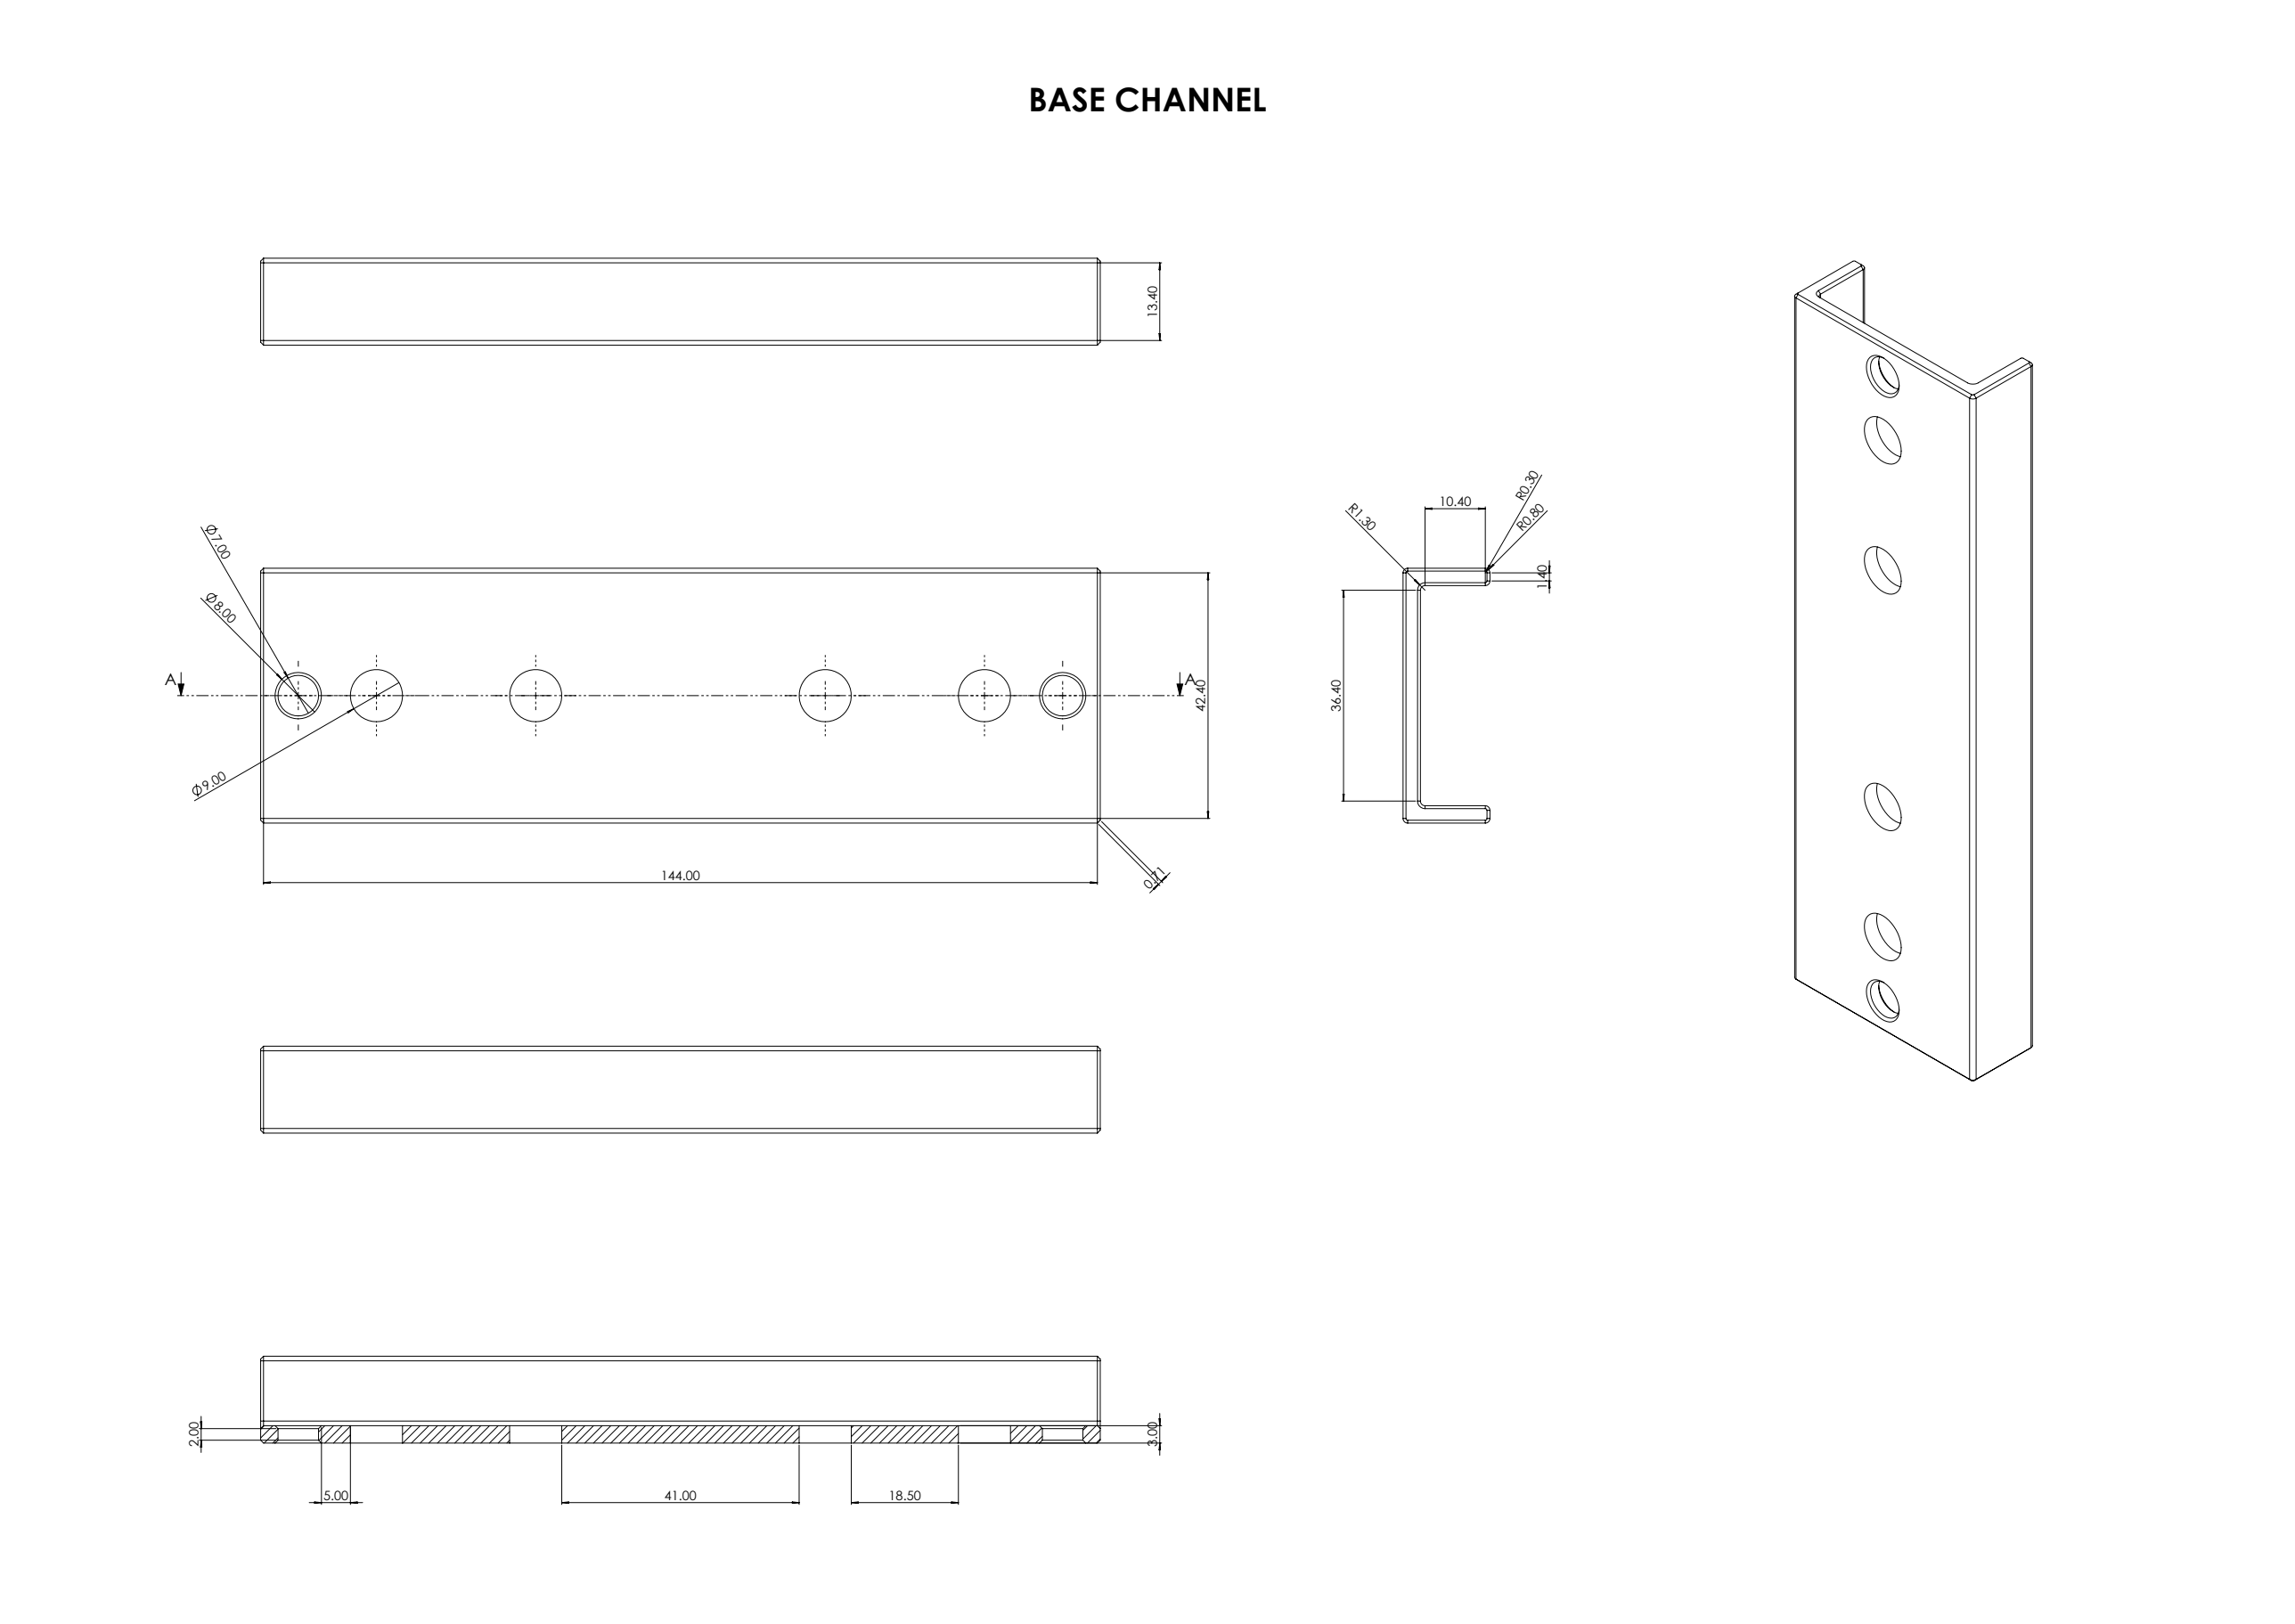
ISO-10303-21;
HEADER;
/* Generated by software containing ST-Developer
 * from STEP Tools, Inc. (www.steptools.com) 
 */

FILE_DESCRIPTION(
/* description */ (''),
/* implementation_level */ '2;1');

FILE_NAME(
/* name */ '14_Base_Channel.step',
/* time_stamp */ '2026-10-26T06:13:19-07:00',
/* author */ (''),
/* organization */ (''),
/* preprocessor_version */ 'ST-DEVELOPER v20.2',
/* originating_system */ 'Autodesk Translation Framework v15.15.0.0',
/* authorisation */ '');

FILE_SCHEMA (('AUTOMOTIVE_DESIGN { 1 0 10303 214 3 1 1 }','TECHNICAL_DATA_PACKAGING'));
ENDSEC;

DATA;
#10=MECHANICAL_DESIGN_GEOMETRIC_PRESENTATION_REPRESENTATION('',(#312),#56639);
#272=SHAPE_REPRESENTATION_RELATIONSHIP('SRR','None',#56760,#292);
#292=ADVANCED_BREP_SHAPE_REPRESENTATION('',(#332),#56634);
#312=STYLED_ITEM('',(#56894),#332);
#332=MANIFOLD_SOLID_BREP('Body1',#16964);
#547=FACE_BOUND('',#3460,.T.);
#548=FACE_BOUND('',#3461,.T.);
#549=FACE_BOUND('',#3462,.T.);
#550=FACE_BOUND('',#3463,.T.);
#551=FACE_BOUND('',#3464,.T.);
#552=FACE_BOUND('',#3465,.T.);
#553=FACE_BOUND('',#3493,.T.);
#554=FACE_BOUND('',#3494,.T.);
#555=FACE_BOUND('',#3495,.T.);
#556=FACE_BOUND('',#3496,.T.);
#557=FACE_BOUND('',#3497,.T.);
#558=FACE_BOUND('',#3498,.T.);
#623=CONICAL_SURFACE('',#18219,3.75,0.785398163397446);
#624=CONICAL_SURFACE('',#18230,3.75,0.785398163397446);
#625=CONICAL_SURFACE('',#18235,0.550000000000001,0.785398163397449);
#626=CONICAL_SURFACE('',#18239,0.550000000000001,0.785398163397449);
#627=CONICAL_SURFACE('',#18243,0.550000000000001,0.785398163397449);
#628=CONICAL_SURFACE('',#18247,1.05,0.785398163397449);
#629=CONICAL_SURFACE('',#18251,1.05,0.785398163397449);
#630=CONICAL_SURFACE('',#18255,0.550000000000001,0.785398163397449);
#631=CONICAL_SURFACE('',#18259,0.550000000000001,0.785398163397449);
#632=CONICAL_SURFACE('',#18263,0.550000000000001,0.785398163397449);
#633=CONICAL_SURFACE('',#18286,0.550000000000001,0.78539816339744);
#634=CONICAL_SURFACE('',#18290,0.550000000000001,0.78539816339744);
#635=CONICAL_SURFACE('',#18294,0.550000000000001,0.78539816339744);
#636=CONICAL_SURFACE('',#18298,1.05,0.78539816339744);
#637=CONICAL_SURFACE('',#18302,1.05,0.78539816339744);
#638=CONICAL_SURFACE('',#18305,0.550000000000001,0.78539816339744);
#639=CONICAL_SURFACE('',#18308,0.550000000000001,0.78539816339744);
#640=CONICAL_SURFACE('',#18311,0.550000000000001,0.78539816339744);
#641=CONICAL_SURFACE('',#18321,3.75,0.785398163397448);
#642=CONICAL_SURFACE('',#18322,3.75,0.785398163397448);
#1132=CIRCLE('',#18220,3.99999999999999);
#1133=CIRCLE('',#18221,3.5);
#1134=CIRCLE('',#18223,3.99999999999999);
#1135=CIRCLE('',#18224,4.5);
#1136=CIRCLE('',#18225,4.5);
#1137=CIRCLE('',#18226,4.5);
#1138=CIRCLE('',#18227,4.5);
#1139=CIRCLE('',#18229,3.5);
#1140=CIRCLE('',#18231,3.5);
#1141=CIRCLE('',#18233,3.5);
#1142=CIRCLE('',#18236,0.8);
#1143=CIRCLE('',#18237,0.300000000000001);
#1144=CIRCLE('',#18240,0.8);
#1145=CIRCLE('',#18241,0.300000000000001);
#1146=CIRCLE('',#18244,0.8);
#1147=CIRCLE('',#18245,0.300000000000001);
#1148=CIRCLE('',#18248,0.8);
#1149=CIRCLE('',#18249,1.3);
#1150=CIRCLE('',#18252,0.8);
#1151=CIRCLE('',#18253,1.3);
#1152=CIRCLE('',#18256,0.8);
#1153=CIRCLE('',#18257,0.300000000000001);
#1154=CIRCLE('',#18260,0.8);
#1155=CIRCLE('',#18261,0.300000000000001);
#1156=CIRCLE('',#18264,0.8);
#1157=CIRCLE('',#18265,0.300000000000001);
#1158=CIRCLE('',#18267,0.8);
#1159=CIRCLE('',#18270,0.8);
#1160=CIRCLE('',#18273,0.8);
#1161=CIRCLE('',#18276,0.8);
#1162=CIRCLE('',#18278,3.99999999999999);
#1163=CIRCLE('',#18279,4.5);
#1164=CIRCLE('',#18280,4.5);
#1165=CIRCLE('',#18281,4.5);
#1166=CIRCLE('',#18282,4.5);
#1167=CIRCLE('',#18283,3.99999999999999);
#1168=CIRCLE('',#18287,0.8);
#1169=CIRCLE('',#18288,0.300000000000001);
#1170=CIRCLE('',#18291,0.8);
#1171=CIRCLE('',#18292,0.300000000000001);
#1172=CIRCLE('',#18295,0.8);
#1173=CIRCLE('',#18296,0.300000000000001);
#1174=CIRCLE('',#18299,0.8);
#1175=CIRCLE('',#18300,1.3);
#1176=CIRCLE('',#18303,1.3);
#1177=CIRCLE('',#18306,0.300000000000001);
#1178=CIRCLE('',#18309,0.300000000000001);
#1179=CIRCLE('',#18312,0.300000000000001);
#1456=CYLINDRICAL_SURFACE('',#18228,3.5);
#1457=CYLINDRICAL_SURFACE('',#18232,3.5);
#1458=CYLINDRICAL_SURFACE('',#18266,0.8);
#1459=CYLINDRICAL_SURFACE('',#18269,0.8);
#1460=CYLINDRICAL_SURFACE('',#18272,0.8);
#1461=CYLINDRICAL_SURFACE('',#18275,0.8);
#1462=CYLINDRICAL_SURFACE('',#18313,0.8);
#1463=CYLINDRICAL_SURFACE('',#18315,0.8);
#1464=CYLINDRICAL_SURFACE('',#18317,0.8);
#1465=CYLINDRICAL_SURFACE('',#18319,0.8);
#1466=CYLINDRICAL_SURFACE('',#18323,4.5);
#1467=CYLINDRICAL_SURFACE('',#18324,4.5);
#1468=CYLINDRICAL_SURFACE('',#18325,4.5);
#1469=CYLINDRICAL_SURFACE('',#18326,4.5);
#2352=FACE_OUTER_BOUND('',#3458,.T.);
#2353=FACE_OUTER_BOUND('',#3459,.T.);
#2354=FACE_OUTER_BOUND('',#3466,.T.);
#2355=FACE_OUTER_BOUND('',#3467,.T.);
#2356=FACE_OUTER_BOUND('',#3468,.T.);
#2357=FACE_OUTER_BOUND('',#3469,.T.);
#2358=FACE_OUTER_BOUND('',#3470,.T.);
#2359=FACE_OUTER_BOUND('',#3471,.T.);
#2360=FACE_OUTER_BOUND('',#3472,.T.);
#2361=FACE_OUTER_BOUND('',#3473,.T.);
#2362=FACE_OUTER_BOUND('',#3474,.T.);
#2363=FACE_OUTER_BOUND('',#3475,.T.);
#2364=FACE_OUTER_BOUND('',#3476,.T.);
#2365=FACE_OUTER_BOUND('',#3477,.T.);
#2366=FACE_OUTER_BOUND('',#3478,.T.);
#2367=FACE_OUTER_BOUND('',#3479,.T.);
#2368=FACE_OUTER_BOUND('',#3480,.T.);
#2369=FACE_OUTER_BOUND('',#3481,.T.);
#2370=FACE_OUTER_BOUND('',#3482,.T.);
#2371=FACE_OUTER_BOUND('',#3483,.T.);
#2372=FACE_OUTER_BOUND('',#3484,.T.);
#2373=FACE_OUTER_BOUND('',#3485,.T.);
#2374=FACE_OUTER_BOUND('',#3486,.T.);
#2375=FACE_OUTER_BOUND('',#3487,.T.);
#2376=FACE_OUTER_BOUND('',#3488,.T.);
#2377=FACE_OUTER_BOUND('',#3489,.T.);
#2378=FACE_OUTER_BOUND('',#3490,.T.);
#2379=FACE_OUTER_BOUND('',#3491,.T.);
#2380=FACE_OUTER_BOUND('',#3492,.T.);
#2381=FACE_OUTER_BOUND('',#3499,.T.);
#2382=FACE_OUTER_BOUND('',#3500,.T.);
#2383=FACE_OUTER_BOUND('',#3501,.T.);
#2384=FACE_OUTER_BOUND('',#3502,.T.);
#2385=FACE_OUTER_BOUND('',#3503,.T.);
#2386=FACE_OUTER_BOUND('',#3504,.T.);
#2387=FACE_OUTER_BOUND('',#3505,.T.);
#2388=FACE_OUTER_BOUND('',#3506,.T.);
#2389=FACE_OUTER_BOUND('',#3507,.T.);
#2390=FACE_OUTER_BOUND('',#3508,.T.);
#2391=FACE_OUTER_BOUND('',#3509,.T.);
#2392=FACE_OUTER_BOUND('',#3510,.T.);
#2393=FACE_OUTER_BOUND('',#3511,.T.);
#2394=FACE_OUTER_BOUND('',#3512,.T.);
#2395=FACE_OUTER_BOUND('',#3513,.T.);
#2396=FACE_OUTER_BOUND('',#3514,.T.);
#2397=FACE_OUTER_BOUND('',#3515,.T.);
#2398=FACE_OUTER_BOUND('',#3516,.T.);
#2399=FACE_OUTER_BOUND('',#3517,.T.);
#2400=FACE_OUTER_BOUND('',#3518,.T.);
#2401=FACE_OUTER_BOUND('',#3519,.T.);
#2402=FACE_OUTER_BOUND('',#3520,.T.);
#2403=FACE_OUTER_BOUND('',#3521,.T.);
#2404=FACE_OUTER_BOUND('',#3522,.T.);
#2405=FACE_OUTER_BOUND('',#3523,.T.);
#2406=FACE_OUTER_BOUND('',#3524,.T.);
#2407=FACE_OUTER_BOUND('',#3525,.T.);
#2408=FACE_OUTER_BOUND('',#3526,.T.);
#2409=FACE_OUTER_BOUND('',#3527,.T.);
#2410=FACE_OUTER_BOUND('',#3528,.T.);
#2411=FACE_OUTER_BOUND('',#3529,.T.);
#3458=EDGE_LOOP('',(#13364,#13365,#13366,#13367));
#3459=EDGE_LOOP('',(#13368,#13369,#13370,#13371));
#3460=EDGE_LOOP('',(#13372));
#3461=EDGE_LOOP('',(#13373));
#3462=EDGE_LOOP('',(#13374));
#3463=EDGE_LOOP('',(#13375));
#3464=EDGE_LOOP('',(#13376));
#3465=EDGE_LOOP('',(#13377));
#3466=EDGE_LOOP('',(#13378,#13379,#13380,#13381));
#3467=EDGE_LOOP('',(#13382,#13383,#13384,#13385));
#3468=EDGE_LOOP('',(#13386,#13387,#13388,#13389));
#3469=EDGE_LOOP('',(#13390,#13391,#13392,#13393));
#3470=EDGE_LOOP('',(#13394,#13395,#13396,#13397));
#3471=EDGE_LOOP('',(#13398,#13399,#13400,#13401));
#3472=EDGE_LOOP('',(#13402,#13403,#13404,#13405));
#3473=EDGE_LOOP('',(#13406,#13407,#13408,#13409));
#3474=EDGE_LOOP('',(#13410,#13411,#13412,#13413));
#3475=EDGE_LOOP('',(#13414,#13415,#13416,#13417));
#3476=EDGE_LOOP('',(#13418,#13419,#13420,#13421));
#3477=EDGE_LOOP('',(#13422,#13423,#13424,#13425));
#3478=EDGE_LOOP('',(#13426,#13427,#13428,#13429));
#3479=EDGE_LOOP('',(#13430,#13431,#13432,#13433));
#3480=EDGE_LOOP('',(#13434,#13435,#13436,#13437));
#3481=EDGE_LOOP('',(#13438,#13439,#13440,#13441));
#3482=EDGE_LOOP('',(#13442,#13443,#13444,#13445));
#3483=EDGE_LOOP('',(#13446,#13447,#13448,#13449));
#3484=EDGE_LOOP('',(#13450,#13451,#13452,#13453));
#3485=EDGE_LOOP('',(#13454,#13455,#13456,#13457));
#3486=EDGE_LOOP('',(#13458,#13459,#13460,#13461));
#3487=EDGE_LOOP('',(#13462,#13463,#13464,#13465));
#3488=EDGE_LOOP('',(#13466,#13467,#13468,#13469));
#3489=EDGE_LOOP('',(#13470,#13471,#13472,#13473));
#3490=EDGE_LOOP('',(#13474,#13475,#13476,#13477));
#3491=EDGE_LOOP('',(#13478,#13479,#13480,#13481));
#3492=EDGE_LOOP('',(#13482,#13483,#13484,#13485));
#3493=EDGE_LOOP('',(#13486));
#3494=EDGE_LOOP('',(#13487));
#3495=EDGE_LOOP('',(#13488));
#3496=EDGE_LOOP('',(#13489));
#3497=EDGE_LOOP('',(#13490));
#3498=EDGE_LOOP('',(#13491));
#3499=EDGE_LOOP('',(#13492,#13493,#13494,#13495,#13496,#13497,#13498,#13499,
#13500,#13501,#13502,#13503,#13504,#13505,#13506,#13507));
#3500=EDGE_LOOP('',(#13508,#13509,#13510,#13511));
#3501=EDGE_LOOP('',(#13512,#13513,#13514,#13515));
#3502=EDGE_LOOP('',(#13516,#13517,#13518,#13519));
#3503=EDGE_LOOP('',(#13520,#13521,#13522,#13523));
#3504=EDGE_LOOP('',(#13524,#13525,#13526,#13527));
#3505=EDGE_LOOP('',(#13528,#13529,#13530,#13531));
#3506=EDGE_LOOP('',(#13532,#13533,#13534,#13535));
#3507=EDGE_LOOP('',(#13536,#13537,#13538,#13539));
#3508=EDGE_LOOP('',(#13540,#13541,#13542,#13543));
#3509=EDGE_LOOP('',(#13544,#13545,#13546,#13547));
#3510=EDGE_LOOP('',(#13548,#13549,#13550,#13551));
#3511=EDGE_LOOP('',(#13552,#13553,#13554,#13555));
#3512=EDGE_LOOP('',(#13556,#13557,#13558,#13559));
#3513=EDGE_LOOP('',(#13560,#13561,#13562,#13563));
#3514=EDGE_LOOP('',(#13564,#13565,#13566,#13567));
#3515=EDGE_LOOP('',(#13568,#13569,#13570,#13571));
#3516=EDGE_LOOP('',(#13572,#13573,#13574,#13575));
#3517=EDGE_LOOP('',(#13576,#13577,#13578,#13579));
#3518=EDGE_LOOP('',(#13580,#13581,#13582,#13583));
#3519=EDGE_LOOP('',(#13584,#13585,#13586,#13587));
#3520=EDGE_LOOP('',(#13588,#13589,#13590,#13591));
#3521=EDGE_LOOP('',(#13592,#13593,#13594,#13595));
#3522=EDGE_LOOP('',(#13596,#13597,#13598,#13599));
#3523=EDGE_LOOP('',(#13600,#13601,#13602,#13603,#13604,#13605,#13606,#13607,
#13608,#13609,#13610,#13611,#13612,#13613,#13614,#13615));
#3524=EDGE_LOOP('',(#13616,#13617,#13618,#13619));
#3525=EDGE_LOOP('',(#13620,#13621,#13622,#13623));
#3526=EDGE_LOOP('',(#13624,#13625,#13626,#13627));
#3527=EDGE_LOOP('',(#13628,#13629,#13630,#13631));
#3528=EDGE_LOOP('',(#13632,#13633,#13634,#13635));
#3529=EDGE_LOOP('',(#13636,#13637,#13638,#13639));
#4425=LINE('',#36461,#5379);
#4426=LINE('',#36466,#5380);
#4427=LINE('',#36468,#5381);
#4428=LINE('',#36470,#5382);
#4429=LINE('',#36471,#5383);
#4430=LINE('',#36485,#5384);
#4431=LINE('',#36488,#5385);
#4432=LINE('',#36493,#5386);
#4433=LINE('',#36497,#5387);
#4434=LINE('',#36499,#5388);
#4435=LINE('',#36501,#5389);
#4436=LINE('',#36502,#5390);
#4437=LINE('',#36507,#5391);
#4438=LINE('',#36512,#5392);
#4439=LINE('',#36513,#5393);
#4440=LINE('',#36514,#5394);
#4441=LINE('',#36519,#5395);
#4442=LINE('',#36524,#5396);
#4443=LINE('',#36525,#5397);
#4444=LINE('',#36526,#5398);
#4445=LINE('',#36531,#5399);
#4446=LINE('',#36536,#5400);
#4447=LINE('',#36537,#5401);
#4448=LINE('',#36538,#5402);
#4449=LINE('',#36542,#5403);
#4450=LINE('',#36546,#5404);
#4451=LINE('',#36547,#5405);
#4452=LINE('',#36552,#5406);
#4453=LINE('',#36557,#5407);
#4454=LINE('',#36558,#5408);
#4455=LINE('',#36559,#5409);
#4456=LINE('',#36564,#5410);
#4457=LINE('',#36569,#5411);
#4458=LINE('',#36570,#5412);
#4459=LINE('',#36571,#5413);
#4460=LINE('',#36576,#5414);
#4461=LINE('',#36581,#5415);
#4462=LINE('',#36582,#5416);
#4463=LINE('',#36583,#5417);
#4464=LINE('',#36589,#5418);
#4465=LINE('',#36593,#5419);
#4466=LINE('',#36594,#5420);
#4467=LINE('',#36597,#5421);
#4468=LINE('',#36601,#5422);
#4469=LINE('',#36602,#5423);
#4470=LINE('',#36605,#5424);
#4471=LINE('',#36609,#5425);
#4472=LINE('',#36610,#5426);
#4473=LINE('',#36613,#5427);
#4474=LINE('',#36617,#5428);
#4475=LINE('',#36618,#5429);
#4476=LINE('',#36634,#5430);
#4477=LINE('',#36636,#5431);
#4478=LINE('',#36637,#5432);
#4479=LINE('',#36642,#5433);
#4480=LINE('',#36647,#5434);
#4481=LINE('',#36648,#5435);
#4482=LINE('',#36649,#5436);
#4483=LINE('',#36654,#5437);
#4484=LINE('',#36659,#5438);
#4485=LINE('',#36660,#5439);
#4486=LINE('',#36661,#5440);
#4487=LINE('',#36666,#5441);
#4488=LINE('',#36671,#5442);
#4489=LINE('',#36672,#5443);
#4490=LINE('',#36673,#5444);
#4491=LINE('',#36677,#5445);
#4492=LINE('',#36681,#5446);
#4493=LINE('',#36682,#5447);
#4494=LINE('',#36685,#5448);
#4495=LINE('',#36689,#5449);
#4496=LINE('',#36690,#5450);
#4497=LINE('',#36693,#5451);
#4498=LINE('',#36697,#5452);
#4499=LINE('',#36698,#5453);
#4500=LINE('',#36701,#5454);
#4501=LINE('',#36705,#5455);
#4502=LINE('',#36706,#5456);
#4503=LINE('',#36710,#5457);
#4504=LINE('',#36712,#5458);
#4505=LINE('',#36714,#5459);
#4506=LINE('',#36716,#5460);
#4507=LINE('',#36718,#5461);
#4508=LINE('',#36720,#5462);
#4509=LINE('',#36724,#5463);
#4510=LINE('',#36726,#5464);
#4511=LINE('',#36728,#5465);
#4512=LINE('',#36730,#5466);
#4513=LINE('',#36732,#5467);
#4514=LINE('',#36734,#5468);
#5379=VECTOR('',#21375,3.75);
#5380=VECTOR('',#21380,10.);
#5381=VECTOR('',#21381,10.);
#5382=VECTOR('',#21382,10.);
#5383=VECTOR('',#21383,10.);
#5384=VECTOR('',#21398,3.5);
#5385=VECTOR('',#21401,3.75);
#5386=VECTOR('',#21408,3.5);
#5387=VECTOR('',#21411,10.);
#5388=VECTOR('',#21412,10.);
#5389=VECTOR('',#21413,10.);
#5390=VECTOR('',#21414,10.);
#5391=VECTOR('',#21419,10.);
#5392=VECTOR('',#21424,10.);
#5393=VECTOR('',#21425,10.);
#5394=VECTOR('',#21426,10.);
#5395=VECTOR('',#21431,10.);
#5396=VECTOR('',#21436,10.);
#5397=VECTOR('',#21437,10.);
#5398=VECTOR('',#21438,10.);
#5399=VECTOR('',#21443,10.);
#5400=VECTOR('',#21448,10.);
#5401=VECTOR('',#21449,10.);
#5402=VECTOR('',#21450,10.);
#5403=VECTOR('',#21455,10.);
#5404=VECTOR('',#21460,10.);
#5405=VECTOR('',#21461,10.);
#5406=VECTOR('',#21466,10.);
#5407=VECTOR('',#21471,10.);
#5408=VECTOR('',#21472,10.);
#5409=VECTOR('',#21473,10.);
#5410=VECTOR('',#21478,10.);
#5411=VECTOR('',#21483,10.);
#5412=VECTOR('',#21484,10.);
#5413=VECTOR('',#21485,10.);
#5414=VECTOR('',#21490,10.);
#5415=VECTOR('',#21495,10.);
#5416=VECTOR('',#21496,10.);
#5417=VECTOR('',#21497,10.);
#5418=VECTOR('',#21506,10.);
#5419=VECTOR('',#21511,10.);
#5420=VECTOR('',#21512,10.);
#5421=VECTOR('',#21515,10.);
#5422=VECTOR('',#21520,10.);
#5423=VECTOR('',#21521,10.);
#5424=VECTOR('',#21524,10.);
#5425=VECTOR('',#21529,10.);
#5426=VECTOR('',#21530,10.);
#5427=VECTOR('',#21533,10.);
#5428=VECTOR('',#21538,10.);
#5429=VECTOR('',#21539,10.);
#5430=VECTOR('',#21556,10.);
#5431=VECTOR('',#21557,10.);
#5432=VECTOR('',#21558,10.);
#5433=VECTOR('',#21563,10.);
#5434=VECTOR('',#21568,10.);
#5435=VECTOR('',#21569,10.);
#5436=VECTOR('',#21570,10.);
#5437=VECTOR('',#21575,10.);
#5438=VECTOR('',#21580,10.);
#5439=VECTOR('',#21581,10.);
#5440=VECTOR('',#21582,10.);
#5441=VECTOR('',#21587,10.);
#5442=VECTOR('',#21592,10.);
#5443=VECTOR('',#21593,10.);
#5444=VECTOR('',#21594,10.);
#5445=VECTOR('',#21599,10.);
#5446=VECTOR('',#21604,10.);
#5447=VECTOR('',#21605,10.);
#5448=VECTOR('',#21608,10.);
#5449=VECTOR('',#21613,10.);
#5450=VECTOR('',#21614,10.);
#5451=VECTOR('',#21617,10.);
#5452=VECTOR('',#21622,10.);
#5453=VECTOR('',#21623,10.);
#5454=VECTOR('',#21626,10.);
#5455=VECTOR('',#21631,10.);
#5456=VECTOR('',#21632,10.);
#5457=VECTOR('',#21639,10.);
#5458=VECTOR('',#21642,10.);
#5459=VECTOR('',#21645,10.);
#5460=VECTOR('',#21648,10.);
#5461=VECTOR('',#21651,10.);
#5462=VECTOR('',#21654,10.);
#5463=VECTOR('',#21661,3.75);
#5464=VECTOR('',#21664,3.75);
#5465=VECTOR('',#21667,4.5);
#5466=VECTOR('',#21670,4.5);
#5467=VECTOR('',#21673,4.5);
#5468=VECTOR('',#21676,4.5);
#7527=VERTEX_POINT('',#36458);
#7528=VERTEX_POINT('',#36460);
#7529=VERTEX_POINT('',#36464);
#7530=VERTEX_POINT('',#36465);
#7531=VERTEX_POINT('',#36467);
#7532=VERTEX_POINT('',#36469);
#7533=VERTEX_POINT('',#36472);
#7534=VERTEX_POINT('',#36474);
#7535=VERTEX_POINT('',#36476);
#7536=VERTEX_POINT('',#36478);
#7537=VERTEX_POINT('',#36480);
#7538=VERTEX_POINT('',#36483);
#7539=VERTEX_POINT('',#36487);
#7540=VERTEX_POINT('',#36491);
#7541=VERTEX_POINT('',#36495);
#7542=VERTEX_POINT('',#36496);
#7543=VERTEX_POINT('',#36498);
#7544=VERTEX_POINT('',#36500);
#7545=VERTEX_POINT('',#36504);
#7546=VERTEX_POINT('',#36506);
#7547=VERTEX_POINT('',#36510);
#7548=VERTEX_POINT('',#36511);
#7549=VERTEX_POINT('',#36516);
#7550=VERTEX_POINT('',#36518);
#7551=VERTEX_POINT('',#36522);
#7552=VERTEX_POINT('',#36523);
#7553=VERTEX_POINT('',#36528);
#7554=VERTEX_POINT('',#36530);
#7555=VERTEX_POINT('',#36534);
#7556=VERTEX_POINT('',#36535);
#7557=VERTEX_POINT('',#36541);
#7558=VERTEX_POINT('',#36545);
#7559=VERTEX_POINT('',#36549);
#7560=VERTEX_POINT('',#36551);
#7561=VERTEX_POINT('',#36555);
#7562=VERTEX_POINT('',#36556);
#7563=VERTEX_POINT('',#36561);
#7564=VERTEX_POINT('',#36563);
#7565=VERTEX_POINT('',#36567);
#7566=VERTEX_POINT('',#36568);
#7567=VERTEX_POINT('',#36573);
#7568=VERTEX_POINT('',#36575);
#7569=VERTEX_POINT('',#36579);
#7570=VERTEX_POINT('',#36580);
#7571=VERTEX_POINT('',#36588);
#7572=VERTEX_POINT('',#36592);
#7573=VERTEX_POINT('',#36596);
#7574=VERTEX_POINT('',#36600);
#7575=VERTEX_POINT('',#36604);
#7576=VERTEX_POINT('',#36608);
#7577=VERTEX_POINT('',#36612);
#7578=VERTEX_POINT('',#36616);
#7579=VERTEX_POINT('',#36619);
#7580=VERTEX_POINT('',#36621);
#7581=VERTEX_POINT('',#36623);
#7582=VERTEX_POINT('',#36625);
#7583=VERTEX_POINT('',#36627);
#7584=VERTEX_POINT('',#36629);
#7585=VERTEX_POINT('',#36633);
#7586=VERTEX_POINT('',#36635);
#7587=VERTEX_POINT('',#36639);
#7588=VERTEX_POINT('',#36641);
#7589=VERTEX_POINT('',#36645);
#7590=VERTEX_POINT('',#36646);
#7591=VERTEX_POINT('',#36651);
#7592=VERTEX_POINT('',#36653);
#7593=VERTEX_POINT('',#36657);
#7594=VERTEX_POINT('',#36658);
#7595=VERTEX_POINT('',#36663);
#7596=VERTEX_POINT('',#36665);
#7597=VERTEX_POINT('',#36669);
#7598=VERTEX_POINT('',#36670);
#7599=VERTEX_POINT('',#36676);
#7600=VERTEX_POINT('',#36680);
#7601=VERTEX_POINT('',#36684);
#7602=VERTEX_POINT('',#36688);
#7603=VERTEX_POINT('',#36692);
#7604=VERTEX_POINT('',#36696);
#7605=VERTEX_POINT('',#36700);
#7606=VERTEX_POINT('',#36704);
#9589=EDGE_CURVE('',#7527,#7527,#1132,.T.);
#9590=EDGE_CURVE('',#7527,#7528,#4425,.T.);
#9591=EDGE_CURVE('',#7528,#7528,#1133,.T.);
#9592=EDGE_CURVE('',#7529,#7530,#4426,.T.);
#9593=EDGE_CURVE('',#7531,#7529,#4427,.T.);
#9594=EDGE_CURVE('',#7532,#7531,#4428,.T.);
#9595=EDGE_CURVE('',#7530,#7532,#4429,.T.);
#9596=EDGE_CURVE('',#7533,#7533,#1134,.T.);
#9597=EDGE_CURVE('',#7534,#7534,#1135,.T.);
#9598=EDGE_CURVE('',#7535,#7535,#1136,.T.);
#9599=EDGE_CURVE('',#7536,#7536,#1137,.T.);
#9600=EDGE_CURVE('',#7537,#7537,#1138,.T.);
#9601=EDGE_CURVE('',#7538,#7538,#1139,.T.);
#9602=EDGE_CURVE('',#7538,#7528,#4430,.T.);
#9603=EDGE_CURVE('',#7533,#7539,#4431,.T.);
#9604=EDGE_CURVE('',#7539,#7539,#1140,.T.);
#9605=EDGE_CURVE('',#7540,#7540,#1141,.T.);
#9606=EDGE_CURVE('',#7540,#7539,#4432,.T.);
#9607=EDGE_CURVE('',#7541,#7542,#4433,.T.);
#9608=EDGE_CURVE('',#7542,#7543,#4434,.T.);
#9609=EDGE_CURVE('',#7543,#7544,#4435,.T.);
#9610=EDGE_CURVE('',#7544,#7541,#4436,.T.);
#9611=EDGE_CURVE('',#7541,#7545,#1142,.T.);
#9612=EDGE_CURVE('',#7545,#7546,#4437,.T.);
#9613=EDGE_CURVE('',#7546,#7542,#1143,.T.);
#9614=EDGE_CURVE('',#7547,#7548,#4438,.T.);
#9615=EDGE_CURVE('',#7548,#7546,#4439,.T.);
#9616=EDGE_CURVE('',#7545,#7547,#4440,.T.);
#9617=EDGE_CURVE('',#7547,#7549,#1144,.T.);
#9618=EDGE_CURVE('',#7549,#7550,#4441,.T.);
#9619=EDGE_CURVE('',#7550,#7548,#1145,.T.);
#9620=EDGE_CURVE('',#7551,#7552,#4442,.T.);
#9621=EDGE_CURVE('',#7552,#7550,#4443,.T.);
#9622=EDGE_CURVE('',#7549,#7551,#4444,.T.);
#9623=EDGE_CURVE('',#7551,#7553,#1146,.T.);
#9624=EDGE_CURVE('',#7553,#7554,#4445,.T.);
#9625=EDGE_CURVE('',#7554,#7552,#1147,.T.);
#9626=EDGE_CURVE('',#7555,#7556,#4446,.T.);
#9627=EDGE_CURVE('',#7556,#7554,#4447,.T.);
#9628=EDGE_CURVE('',#7553,#7555,#4448,.T.);
#9629=EDGE_CURVE('',#7555,#7529,#1148,.T.);
#9630=EDGE_CURVE('',#7529,#7557,#4449,.T.);
#9631=EDGE_CURVE('',#7557,#7556,#1149,.T.);
#9632=EDGE_CURVE('',#7530,#7558,#4450,.T.);
#9633=EDGE_CURVE('',#7558,#7557,#4451,.T.);
#9634=EDGE_CURVE('',#7530,#7559,#1150,.T.);
#9635=EDGE_CURVE('',#7559,#7560,#4452,.T.);
#9636=EDGE_CURVE('',#7560,#7558,#1151,.T.);
#9637=EDGE_CURVE('',#7561,#7562,#4453,.T.);
#9638=EDGE_CURVE('',#7562,#7560,#4454,.T.);
#9639=EDGE_CURVE('',#7559,#7561,#4455,.T.);
#9640=EDGE_CURVE('',#7561,#7563,#1152,.T.);
#9641=EDGE_CURVE('',#7563,#7564,#4456,.T.);
#9642=EDGE_CURVE('',#7564,#7562,#1153,.T.);
#9643=EDGE_CURVE('',#7565,#7566,#4457,.T.);
#9644=EDGE_CURVE('',#7566,#7564,#4458,.T.);
#9645=EDGE_CURVE('',#7563,#7565,#4459,.T.);
#9646=EDGE_CURVE('',#7565,#7567,#1154,.T.);
#9647=EDGE_CURVE('',#7567,#7568,#4460,.T.);
#9648=EDGE_CURVE('',#7568,#7566,#1155,.T.);
#9649=EDGE_CURVE('',#7569,#7570,#4461,.T.);
#9650=EDGE_CURVE('',#7570,#7568,#4462,.T.);
#9651=EDGE_CURVE('',#7567,#7569,#4463,.T.);
#9652=EDGE_CURVE('',#7569,#7544,#1156,.T.);
#9653=EDGE_CURVE('',#7543,#7570,#1157,.T.);
#9654=EDGE_CURVE('',#7555,#7571,#4464,.T.);
#9655=EDGE_CURVE('',#7531,#7571,#1158,.T.);
#9656=EDGE_CURVE('',#7572,#7553,#4465,.T.);
#9657=EDGE_CURVE('',#7571,#7572,#4466,.T.);
#9658=EDGE_CURVE('',#7551,#7573,#4467,.T.);
#9659=EDGE_CURVE('',#7572,#7573,#1159,.T.);
#9660=EDGE_CURVE('',#7574,#7549,#4468,.T.);
#9661=EDGE_CURVE('',#7573,#7574,#4469,.T.);
#9662=EDGE_CURVE('',#7547,#7575,#4470,.T.);
#9663=EDGE_CURVE('',#7574,#7575,#1160,.T.);
#9664=EDGE_CURVE('',#7576,#7545,#4471,.T.);
#9665=EDGE_CURVE('',#7575,#7576,#4472,.T.);
#9666=EDGE_CURVE('',#7541,#7577,#4473,.T.);
#9667=EDGE_CURVE('',#7576,#7577,#1161,.T.);
#9668=EDGE_CURVE('',#7578,#7544,#4474,.T.);
#9669=EDGE_CURVE('',#7577,#7578,#4475,.T.);
#9670=EDGE_CURVE('',#7579,#7579,#1162,.T.);
#9671=EDGE_CURVE('',#7580,#7580,#1163,.T.);
#9672=EDGE_CURVE('',#7581,#7581,#1164,.T.);
#9673=EDGE_CURVE('',#7582,#7582,#1165,.T.);
#9674=EDGE_CURVE('',#7583,#7583,#1166,.T.);
#9675=EDGE_CURVE('',#7584,#7584,#1167,.T.);
#9676=EDGE_CURVE('',#7578,#7585,#4476,.T.);
#9677=EDGE_CURVE('',#7585,#7586,#4477,.T.);
#9678=EDGE_CURVE('',#7586,#7577,#4478,.T.);
#9679=EDGE_CURVE('',#7578,#7587,#1168,.T.);
#9680=EDGE_CURVE('',#7587,#7588,#4479,.T.);
#9681=EDGE_CURVE('',#7588,#7585,#1169,.T.);
#9682=EDGE_CURVE('',#7589,#7590,#4480,.T.);
#9683=EDGE_CURVE('',#7590,#7588,#4481,.T.);
#9684=EDGE_CURVE('',#7587,#7589,#4482,.T.);
#9685=EDGE_CURVE('',#7589,#7591,#1170,.T.);
#9686=EDGE_CURVE('',#7591,#7592,#4483,.T.);
#9687=EDGE_CURVE('',#7592,#7590,#1171,.T.);
#9688=EDGE_CURVE('',#7593,#7594,#4484,.T.);
#9689=EDGE_CURVE('',#7594,#7592,#4485,.T.);
#9690=EDGE_CURVE('',#7591,#7593,#4486,.T.);
#9691=EDGE_CURVE('',#7593,#7595,#1172,.T.);
#9692=EDGE_CURVE('',#7595,#7596,#4487,.T.);
#9693=EDGE_CURVE('',#7596,#7594,#1173,.T.);
#9694=EDGE_CURVE('',#7597,#7598,#4488,.T.);
#9695=EDGE_CURVE('',#7598,#7596,#4489,.T.);
#9696=EDGE_CURVE('',#7595,#7597,#4490,.T.);
#9697=EDGE_CURVE('',#7597,#7532,#1174,.T.);
#9698=EDGE_CURVE('',#7532,#7599,#4491,.T.);
#9699=EDGE_CURVE('',#7599,#7598,#1175,.T.);
#9700=EDGE_CURVE('',#7531,#7600,#4492,.T.);
#9701=EDGE_CURVE('',#7600,#7599,#4493,.T.);
#9702=EDGE_CURVE('',#7571,#7601,#4494,.T.);
#9703=EDGE_CURVE('',#7601,#7600,#1176,.T.);
#9704=EDGE_CURVE('',#7572,#7602,#4495,.T.);
#9705=EDGE_CURVE('',#7602,#7601,#4496,.T.);
#9706=EDGE_CURVE('',#7573,#7603,#4497,.T.);
#9707=EDGE_CURVE('',#7603,#7602,#1177,.T.);
#9708=EDGE_CURVE('',#7574,#7604,#4498,.T.);
#9709=EDGE_CURVE('',#7604,#7603,#4499,.T.);
#9710=EDGE_CURVE('',#7575,#7605,#4500,.T.);
#9711=EDGE_CURVE('',#7605,#7604,#1178,.T.);
#9712=EDGE_CURVE('',#7576,#7606,#4501,.T.);
#9713=EDGE_CURVE('',#7606,#7605,#4502,.T.);
#9714=EDGE_CURVE('',#7586,#7606,#1179,.T.);
#9715=EDGE_CURVE('',#7597,#7559,#4503,.T.);
#9716=EDGE_CURVE('',#7561,#7595,#4504,.T.);
#9717=EDGE_CURVE('',#7593,#7563,#4505,.T.);
#9718=EDGE_CURVE('',#7565,#7591,#4506,.T.);
#9719=EDGE_CURVE('',#7589,#7567,#4507,.T.);
#9720=EDGE_CURVE('',#7569,#7587,#4508,.T.);
#9721=EDGE_CURVE('',#7584,#7540,#4509,.T.);
#9722=EDGE_CURVE('',#7579,#7538,#4510,.T.);
#9723=EDGE_CURVE('',#7580,#7537,#4511,.T.);
#9724=EDGE_CURVE('',#7581,#7536,#4512,.T.);
#9725=EDGE_CURVE('',#7582,#7535,#4513,.T.);
#9726=EDGE_CURVE('',#7583,#7534,#4514,.T.);
#13364=ORIENTED_EDGE('',*,*,#9589,.T.);
#13365=ORIENTED_EDGE('',*,*,#9590,.T.);
#13366=ORIENTED_EDGE('',*,*,#9591,.T.);
#13367=ORIENTED_EDGE('',*,*,#9590,.F.);
#13368=ORIENTED_EDGE('',*,*,#9592,.F.);
#13369=ORIENTED_EDGE('',*,*,#9593,.F.);
#13370=ORIENTED_EDGE('',*,*,#9594,.F.);
#13371=ORIENTED_EDGE('',*,*,#9595,.F.);
#13372=ORIENTED_EDGE('',*,*,#9596,.F.);
#13373=ORIENTED_EDGE('',*,*,#9597,.T.);
#13374=ORIENTED_EDGE('',*,*,#9598,.T.);
#13375=ORIENTED_EDGE('',*,*,#9599,.T.);
#13376=ORIENTED_EDGE('',*,*,#9600,.T.);
#13377=ORIENTED_EDGE('',*,*,#9589,.F.);
#13378=ORIENTED_EDGE('',*,*,#9601,.F.);
#13379=ORIENTED_EDGE('',*,*,#9602,.T.);
#13380=ORIENTED_EDGE('',*,*,#9591,.F.);
#13381=ORIENTED_EDGE('',*,*,#9602,.F.);
#13382=ORIENTED_EDGE('',*,*,#9596,.T.);
#13383=ORIENTED_EDGE('',*,*,#9603,.T.);
#13384=ORIENTED_EDGE('',*,*,#9604,.T.);
#13385=ORIENTED_EDGE('',*,*,#9603,.F.);
#13386=ORIENTED_EDGE('',*,*,#9605,.F.);
#13387=ORIENTED_EDGE('',*,*,#9606,.T.);
#13388=ORIENTED_EDGE('',*,*,#9604,.F.);
#13389=ORIENTED_EDGE('',*,*,#9606,.F.);
#13390=ORIENTED_EDGE('',*,*,#9607,.T.);
#13391=ORIENTED_EDGE('',*,*,#9608,.T.);
#13392=ORIENTED_EDGE('',*,*,#9609,.T.);
#13393=ORIENTED_EDGE('',*,*,#9610,.T.);
#13394=ORIENTED_EDGE('',*,*,#9607,.F.);
#13395=ORIENTED_EDGE('',*,*,#9611,.T.);
#13396=ORIENTED_EDGE('',*,*,#9612,.T.);
#13397=ORIENTED_EDGE('',*,*,#9613,.T.);
#13398=ORIENTED_EDGE('',*,*,#9614,.T.);
#13399=ORIENTED_EDGE('',*,*,#9615,.T.);
#13400=ORIENTED_EDGE('',*,*,#9612,.F.);
#13401=ORIENTED_EDGE('',*,*,#9616,.T.);
#13402=ORIENTED_EDGE('',*,*,#9614,.F.);
#13403=ORIENTED_EDGE('',*,*,#9617,.T.);
#13404=ORIENTED_EDGE('',*,*,#9618,.T.);
#13405=ORIENTED_EDGE('',*,*,#9619,.T.);
#13406=ORIENTED_EDGE('',*,*,#9620,.T.);
#13407=ORIENTED_EDGE('',*,*,#9621,.T.);
#13408=ORIENTED_EDGE('',*,*,#9618,.F.);
#13409=ORIENTED_EDGE('',*,*,#9622,.T.);
#13410=ORIENTED_EDGE('',*,*,#9620,.F.);
#13411=ORIENTED_EDGE('',*,*,#9623,.T.);
#13412=ORIENTED_EDGE('',*,*,#9624,.T.);
#13413=ORIENTED_EDGE('',*,*,#9625,.T.);
#13414=ORIENTED_EDGE('',*,*,#9626,.T.);
#13415=ORIENTED_EDGE('',*,*,#9627,.T.);
#13416=ORIENTED_EDGE('',*,*,#9624,.F.);
#13417=ORIENTED_EDGE('',*,*,#9628,.T.);
#13418=ORIENTED_EDGE('',*,*,#9626,.F.);
#13419=ORIENTED_EDGE('',*,*,#9629,.T.);
#13420=ORIENTED_EDGE('',*,*,#9630,.T.);
#13421=ORIENTED_EDGE('',*,*,#9631,.T.);
#13422=ORIENTED_EDGE('',*,*,#9632,.T.);
#13423=ORIENTED_EDGE('',*,*,#9633,.T.);
#13424=ORIENTED_EDGE('',*,*,#9630,.F.);
#13425=ORIENTED_EDGE('',*,*,#9592,.T.);
#13426=ORIENTED_EDGE('',*,*,#9632,.F.);
#13427=ORIENTED_EDGE('',*,*,#9634,.T.);
#13428=ORIENTED_EDGE('',*,*,#9635,.T.);
#13429=ORIENTED_EDGE('',*,*,#9636,.T.);
#13430=ORIENTED_EDGE('',*,*,#9637,.T.);
#13431=ORIENTED_EDGE('',*,*,#9638,.T.);
#13432=ORIENTED_EDGE('',*,*,#9635,.F.);
#13433=ORIENTED_EDGE('',*,*,#9639,.T.);
#13434=ORIENTED_EDGE('',*,*,#9637,.F.);
#13435=ORIENTED_EDGE('',*,*,#9640,.T.);
#13436=ORIENTED_EDGE('',*,*,#9641,.T.);
#13437=ORIENTED_EDGE('',*,*,#9642,.T.);
#13438=ORIENTED_EDGE('',*,*,#9643,.T.);
#13439=ORIENTED_EDGE('',*,*,#9644,.T.);
#13440=ORIENTED_EDGE('',*,*,#9641,.F.);
#13441=ORIENTED_EDGE('',*,*,#9645,.T.);
#13442=ORIENTED_EDGE('',*,*,#9643,.F.);
#13443=ORIENTED_EDGE('',*,*,#9646,.T.);
#13444=ORIENTED_EDGE('',*,*,#9647,.T.);
#13445=ORIENTED_EDGE('',*,*,#9648,.T.);
#13446=ORIENTED_EDGE('',*,*,#9649,.T.);
#13447=ORIENTED_EDGE('',*,*,#9650,.T.);
#13448=ORIENTED_EDGE('',*,*,#9647,.F.);
#13449=ORIENTED_EDGE('',*,*,#9651,.T.);
#13450=ORIENTED_EDGE('',*,*,#9649,.F.);
#13451=ORIENTED_EDGE('',*,*,#9652,.T.);
#13452=ORIENTED_EDGE('',*,*,#9609,.F.);
#13453=ORIENTED_EDGE('',*,*,#9653,.T.);
#13454=ORIENTED_EDGE('',*,*,#9629,.F.);
#13455=ORIENTED_EDGE('',*,*,#9654,.T.);
#13456=ORIENTED_EDGE('',*,*,#9655,.F.);
#13457=ORIENTED_EDGE('',*,*,#9593,.T.);
#13458=ORIENTED_EDGE('',*,*,#9628,.F.);
#13459=ORIENTED_EDGE('',*,*,#9656,.F.);
#13460=ORIENTED_EDGE('',*,*,#9657,.F.);
#13461=ORIENTED_EDGE('',*,*,#9654,.F.);
#13462=ORIENTED_EDGE('',*,*,#9623,.F.);
#13463=ORIENTED_EDGE('',*,*,#9658,.T.);
#13464=ORIENTED_EDGE('',*,*,#9659,.F.);
#13465=ORIENTED_EDGE('',*,*,#9656,.T.);
#13466=ORIENTED_EDGE('',*,*,#9622,.F.);
#13467=ORIENTED_EDGE('',*,*,#9660,.F.);
#13468=ORIENTED_EDGE('',*,*,#9661,.F.);
#13469=ORIENTED_EDGE('',*,*,#9658,.F.);
#13470=ORIENTED_EDGE('',*,*,#9617,.F.);
#13471=ORIENTED_EDGE('',*,*,#9662,.T.);
#13472=ORIENTED_EDGE('',*,*,#9663,.F.);
#13473=ORIENTED_EDGE('',*,*,#9660,.T.);
#13474=ORIENTED_EDGE('',*,*,#9616,.F.);
#13475=ORIENTED_EDGE('',*,*,#9664,.F.);
#13476=ORIENTED_EDGE('',*,*,#9665,.F.);
#13477=ORIENTED_EDGE('',*,*,#9662,.F.);
#13478=ORIENTED_EDGE('',*,*,#9611,.F.);
#13479=ORIENTED_EDGE('',*,*,#9666,.T.);
#13480=ORIENTED_EDGE('',*,*,#9667,.F.);
#13481=ORIENTED_EDGE('',*,*,#9664,.T.);
#13482=ORIENTED_EDGE('',*,*,#9610,.F.);
#13483=ORIENTED_EDGE('',*,*,#9668,.F.);
#13484=ORIENTED_EDGE('',*,*,#9669,.F.);
#13485=ORIENTED_EDGE('',*,*,#9666,.F.);
#13486=ORIENTED_EDGE('',*,*,#9670,.F.);
#13487=ORIENTED_EDGE('',*,*,#9671,.T.);
#13488=ORIENTED_EDGE('',*,*,#9672,.T.);
#13489=ORIENTED_EDGE('',*,*,#9673,.T.);
#13490=ORIENTED_EDGE('',*,*,#9674,.T.);
#13491=ORIENTED_EDGE('',*,*,#9675,.F.);
#13492=ORIENTED_EDGE('',*,*,#9608,.F.);
#13493=ORIENTED_EDGE('',*,*,#9613,.F.);
#13494=ORIENTED_EDGE('',*,*,#9615,.F.);
#13495=ORIENTED_EDGE('',*,*,#9619,.F.);
#13496=ORIENTED_EDGE('',*,*,#9621,.F.);
#13497=ORIENTED_EDGE('',*,*,#9625,.F.);
#13498=ORIENTED_EDGE('',*,*,#9627,.F.);
#13499=ORIENTED_EDGE('',*,*,#9631,.F.);
#13500=ORIENTED_EDGE('',*,*,#9633,.F.);
#13501=ORIENTED_EDGE('',*,*,#9636,.F.);
#13502=ORIENTED_EDGE('',*,*,#9638,.F.);
#13503=ORIENTED_EDGE('',*,*,#9642,.F.);
#13504=ORIENTED_EDGE('',*,*,#9644,.F.);
#13505=ORIENTED_EDGE('',*,*,#9648,.F.);
#13506=ORIENTED_EDGE('',*,*,#9650,.F.);
#13507=ORIENTED_EDGE('',*,*,#9653,.F.);
#13508=ORIENTED_EDGE('',*,*,#9676,.T.);
#13509=ORIENTED_EDGE('',*,*,#9677,.T.);
#13510=ORIENTED_EDGE('',*,*,#9678,.T.);
#13511=ORIENTED_EDGE('',*,*,#9669,.T.);
#13512=ORIENTED_EDGE('',*,*,#9676,.F.);
#13513=ORIENTED_EDGE('',*,*,#9679,.T.);
#13514=ORIENTED_EDGE('',*,*,#9680,.T.);
#13515=ORIENTED_EDGE('',*,*,#9681,.T.);
#13516=ORIENTED_EDGE('',*,*,#9682,.T.);
#13517=ORIENTED_EDGE('',*,*,#9683,.T.);
#13518=ORIENTED_EDGE('',*,*,#9680,.F.);
#13519=ORIENTED_EDGE('',*,*,#9684,.T.);
#13520=ORIENTED_EDGE('',*,*,#9682,.F.);
#13521=ORIENTED_EDGE('',*,*,#9685,.T.);
#13522=ORIENTED_EDGE('',*,*,#9686,.T.);
#13523=ORIENTED_EDGE('',*,*,#9687,.T.);
#13524=ORIENTED_EDGE('',*,*,#9688,.T.);
#13525=ORIENTED_EDGE('',*,*,#9689,.T.);
#13526=ORIENTED_EDGE('',*,*,#9686,.F.);
#13527=ORIENTED_EDGE('',*,*,#9690,.T.);
#13528=ORIENTED_EDGE('',*,*,#9688,.F.);
#13529=ORIENTED_EDGE('',*,*,#9691,.T.);
#13530=ORIENTED_EDGE('',*,*,#9692,.T.);
#13531=ORIENTED_EDGE('',*,*,#9693,.T.);
#13532=ORIENTED_EDGE('',*,*,#9694,.T.);
#13533=ORIENTED_EDGE('',*,*,#9695,.T.);
#13534=ORIENTED_EDGE('',*,*,#9692,.F.);
#13535=ORIENTED_EDGE('',*,*,#9696,.T.);
#13536=ORIENTED_EDGE('',*,*,#9694,.F.);
#13537=ORIENTED_EDGE('',*,*,#9697,.T.);
#13538=ORIENTED_EDGE('',*,*,#9698,.T.);
#13539=ORIENTED_EDGE('',*,*,#9699,.T.);
#13540=ORIENTED_EDGE('',*,*,#9700,.T.);
#13541=ORIENTED_EDGE('',*,*,#9701,.T.);
#13542=ORIENTED_EDGE('',*,*,#9698,.F.);
#13543=ORIENTED_EDGE('',*,*,#9594,.T.);
#13544=ORIENTED_EDGE('',*,*,#9700,.F.);
#13545=ORIENTED_EDGE('',*,*,#9655,.T.);
#13546=ORIENTED_EDGE('',*,*,#9702,.T.);
#13547=ORIENTED_EDGE('',*,*,#9703,.T.);
#13548=ORIENTED_EDGE('',*,*,#9704,.T.);
#13549=ORIENTED_EDGE('',*,*,#9705,.T.);
#13550=ORIENTED_EDGE('',*,*,#9702,.F.);
#13551=ORIENTED_EDGE('',*,*,#9657,.T.);
#13552=ORIENTED_EDGE('',*,*,#9704,.F.);
#13553=ORIENTED_EDGE('',*,*,#9659,.T.);
#13554=ORIENTED_EDGE('',*,*,#9706,.T.);
#13555=ORIENTED_EDGE('',*,*,#9707,.T.);
#13556=ORIENTED_EDGE('',*,*,#9708,.T.);
#13557=ORIENTED_EDGE('',*,*,#9709,.T.);
#13558=ORIENTED_EDGE('',*,*,#9706,.F.);
#13559=ORIENTED_EDGE('',*,*,#9661,.T.);
#13560=ORIENTED_EDGE('',*,*,#9708,.F.);
#13561=ORIENTED_EDGE('',*,*,#9663,.T.);
#13562=ORIENTED_EDGE('',*,*,#9710,.T.);
#13563=ORIENTED_EDGE('',*,*,#9711,.T.);
#13564=ORIENTED_EDGE('',*,*,#9712,.T.);
#13565=ORIENTED_EDGE('',*,*,#9713,.T.);
#13566=ORIENTED_EDGE('',*,*,#9710,.F.);
#13567=ORIENTED_EDGE('',*,*,#9665,.T.);
#13568=ORIENTED_EDGE('',*,*,#9712,.F.);
#13569=ORIENTED_EDGE('',*,*,#9667,.T.);
#13570=ORIENTED_EDGE('',*,*,#9678,.F.);
#13571=ORIENTED_EDGE('',*,*,#9714,.T.);
#13572=ORIENTED_EDGE('',*,*,#9634,.F.);
#13573=ORIENTED_EDGE('',*,*,#9595,.T.);
#13574=ORIENTED_EDGE('',*,*,#9697,.F.);
#13575=ORIENTED_EDGE('',*,*,#9715,.T.);
#13576=ORIENTED_EDGE('',*,*,#9639,.F.);
#13577=ORIENTED_EDGE('',*,*,#9715,.F.);
#13578=ORIENTED_EDGE('',*,*,#9696,.F.);
#13579=ORIENTED_EDGE('',*,*,#9716,.F.);
#13580=ORIENTED_EDGE('',*,*,#9640,.F.);
#13581=ORIENTED_EDGE('',*,*,#9716,.T.);
#13582=ORIENTED_EDGE('',*,*,#9691,.F.);
#13583=ORIENTED_EDGE('',*,*,#9717,.T.);
#13584=ORIENTED_EDGE('',*,*,#9645,.F.);
#13585=ORIENTED_EDGE('',*,*,#9717,.F.);
#13586=ORIENTED_EDGE('',*,*,#9690,.F.);
#13587=ORIENTED_EDGE('',*,*,#9718,.F.);
#13588=ORIENTED_EDGE('',*,*,#9646,.F.);
#13589=ORIENTED_EDGE('',*,*,#9718,.T.);
#13590=ORIENTED_EDGE('',*,*,#9685,.F.);
#13591=ORIENTED_EDGE('',*,*,#9719,.T.);
#13592=ORIENTED_EDGE('',*,*,#9651,.F.);
#13593=ORIENTED_EDGE('',*,*,#9719,.F.);
#13594=ORIENTED_EDGE('',*,*,#9684,.F.);
#13595=ORIENTED_EDGE('',*,*,#9720,.F.);
#13596=ORIENTED_EDGE('',*,*,#9652,.F.);
#13597=ORIENTED_EDGE('',*,*,#9720,.T.);
#13598=ORIENTED_EDGE('',*,*,#9679,.F.);
#13599=ORIENTED_EDGE('',*,*,#9668,.T.);
#13600=ORIENTED_EDGE('',*,*,#9677,.F.);
#13601=ORIENTED_EDGE('',*,*,#9681,.F.);
#13602=ORIENTED_EDGE('',*,*,#9683,.F.);
#13603=ORIENTED_EDGE('',*,*,#9687,.F.);
#13604=ORIENTED_EDGE('',*,*,#9689,.F.);
#13605=ORIENTED_EDGE('',*,*,#9693,.F.);
#13606=ORIENTED_EDGE('',*,*,#9695,.F.);
#13607=ORIENTED_EDGE('',*,*,#9699,.F.);
#13608=ORIENTED_EDGE('',*,*,#9701,.F.);
#13609=ORIENTED_EDGE('',*,*,#9703,.F.);
#13610=ORIENTED_EDGE('',*,*,#9705,.F.);
#13611=ORIENTED_EDGE('',*,*,#9707,.F.);
#13612=ORIENTED_EDGE('',*,*,#9709,.F.);
#13613=ORIENTED_EDGE('',*,*,#9711,.F.);
#13614=ORIENTED_EDGE('',*,*,#9713,.F.);
#13615=ORIENTED_EDGE('',*,*,#9714,.F.);
#13616=ORIENTED_EDGE('',*,*,#9675,.T.);
#13617=ORIENTED_EDGE('',*,*,#9721,.T.);
#13618=ORIENTED_EDGE('',*,*,#9605,.T.);
#13619=ORIENTED_EDGE('',*,*,#9721,.F.);
#13620=ORIENTED_EDGE('',*,*,#9670,.T.);
#13621=ORIENTED_EDGE('',*,*,#9722,.T.);
#13622=ORIENTED_EDGE('',*,*,#9601,.T.);
#13623=ORIENTED_EDGE('',*,*,#9722,.F.);
#13624=ORIENTED_EDGE('',*,*,#9671,.F.);
#13625=ORIENTED_EDGE('',*,*,#9723,.T.);
#13626=ORIENTED_EDGE('',*,*,#9600,.F.);
#13627=ORIENTED_EDGE('',*,*,#9723,.F.);
#13628=ORIENTED_EDGE('',*,*,#9672,.F.);
#13629=ORIENTED_EDGE('',*,*,#9724,.T.);
#13630=ORIENTED_EDGE('',*,*,#9599,.F.);
#13631=ORIENTED_EDGE('',*,*,#9724,.F.);
#13632=ORIENTED_EDGE('',*,*,#9673,.F.);
#13633=ORIENTED_EDGE('',*,*,#9725,.T.);
#13634=ORIENTED_EDGE('',*,*,#9598,.F.);
#13635=ORIENTED_EDGE('',*,*,#9725,.F.);
#13636=ORIENTED_EDGE('',*,*,#9674,.F.);
#13637=ORIENTED_EDGE('',*,*,#9726,.T.);
#13638=ORIENTED_EDGE('',*,*,#9597,.F.);
#13639=ORIENTED_EDGE('',*,*,#9726,.F.);
#15906=PLANE('',#18222);
#15907=PLANE('',#18234);
#15908=PLANE('',#18238);
#15909=PLANE('',#18242);
#15910=PLANE('',#18246);
#15911=PLANE('',#18250);
#15912=PLANE('',#18254);
#15913=PLANE('',#18258);
#15914=PLANE('',#18262);
#15915=PLANE('',#18268);
#15916=PLANE('',#18271);
#15917=PLANE('',#18274);
#15918=PLANE('',#18277);
#15919=PLANE('',#18284);
#15920=PLANE('',#18285);
#15921=PLANE('',#18289);
#15922=PLANE('',#18293);
#15923=PLANE('',#18297);
#15924=PLANE('',#18301);
#15925=PLANE('',#18304);
#15926=PLANE('',#18307);
#15927=PLANE('',#18310);
#15928=PLANE('',#18314);
#15929=PLANE('',#18316);
#15930=PLANE('',#18318);
#15931=PLANE('',#18320);
#16523=ADVANCED_FACE('',(#2352),#623,.F.);
#16524=ADVANCED_FACE('',(#2353,#547,#548,#549,#550,#551,#552),#15906,.T.);
#16525=ADVANCED_FACE('',(#2354),#1456,.F.);
#16526=ADVANCED_FACE('',(#2355),#624,.F.);
#16527=ADVANCED_FACE('',(#2356),#1457,.F.);
#16528=ADVANCED_FACE('',(#2357),#15907,.T.);
#16529=ADVANCED_FACE('',(#2358),#625,.T.);
#16530=ADVANCED_FACE('',(#2359),#15908,.T.);
#16531=ADVANCED_FACE('',(#2360),#626,.T.);
#16532=ADVANCED_FACE('',(#2361),#15909,.T.);
#16533=ADVANCED_FACE('',(#2362),#627,.T.);
#16534=ADVANCED_FACE('',(#2363),#15910,.T.);
#16535=ADVANCED_FACE('',(#2364),#628,.F.);
#16536=ADVANCED_FACE('',(#2365),#15911,.T.);
#16537=ADVANCED_FACE('',(#2366),#629,.F.);
#16538=ADVANCED_FACE('',(#2367),#15912,.T.);
#16539=ADVANCED_FACE('',(#2368),#630,.T.);
#16540=ADVANCED_FACE('',(#2369),#15913,.T.);
#16541=ADVANCED_FACE('',(#2370),#631,.T.);
#16542=ADVANCED_FACE('',(#2371),#15914,.T.);
#16543=ADVANCED_FACE('',(#2372),#632,.T.);
#16544=ADVANCED_FACE('',(#2373),#1458,.F.);
#16545=ADVANCED_FACE('',(#2374),#15915,.T.);
#16546=ADVANCED_FACE('',(#2375),#1459,.T.);
#16547=ADVANCED_FACE('',(#2376),#15916,.T.);
#16548=ADVANCED_FACE('',(#2377),#1460,.T.);
#16549=ADVANCED_FACE('',(#2378),#15917,.T.);
#16550=ADVANCED_FACE('',(#2379),#1461,.T.);
#16551=ADVANCED_FACE('',(#2380,#553,#554,#555,#556,#557,#558),#15918,.T.);
#16552=ADVANCED_FACE('',(#2381),#15919,.F.);
#16553=ADVANCED_FACE('',(#2382),#15920,.T.);
#16554=ADVANCED_FACE('',(#2383),#633,.T.);
#16555=ADVANCED_FACE('',(#2384),#15921,.T.);
#16556=ADVANCED_FACE('',(#2385),#634,.T.);
#16557=ADVANCED_FACE('',(#2386),#15922,.T.);
#16558=ADVANCED_FACE('',(#2387),#635,.T.);
#16559=ADVANCED_FACE('',(#2388),#15923,.T.);
#16560=ADVANCED_FACE('',(#2389),#636,.F.);
#16561=ADVANCED_FACE('',(#2390),#15924,.T.);
#16562=ADVANCED_FACE('',(#2391),#637,.F.);
#16563=ADVANCED_FACE('',(#2392),#15925,.T.);
#16564=ADVANCED_FACE('',(#2393),#638,.T.);
#16565=ADVANCED_FACE('',(#2394),#15926,.T.);
#16566=ADVANCED_FACE('',(#2395),#639,.T.);
#16567=ADVANCED_FACE('',(#2396),#15927,.T.);
#16568=ADVANCED_FACE('',(#2397),#640,.T.);
#16569=ADVANCED_FACE('',(#2398),#1462,.F.);
#16570=ADVANCED_FACE('',(#2399),#15928,.T.);
#16571=ADVANCED_FACE('',(#2400),#1463,.T.);
#16572=ADVANCED_FACE('',(#2401),#15929,.T.);
#16573=ADVANCED_FACE('',(#2402),#1464,.T.);
#16574=ADVANCED_FACE('',(#2403),#15930,.T.);
#16575=ADVANCED_FACE('',(#2404),#1465,.T.);
#16576=ADVANCED_FACE('',(#2405),#15931,.T.);
#16577=ADVANCED_FACE('',(#2406),#641,.F.);
#16578=ADVANCED_FACE('',(#2407),#642,.F.);
#16579=ADVANCED_FACE('',(#2408),#1466,.F.);
#16580=ADVANCED_FACE('',(#2409),#1467,.F.);
#16581=ADVANCED_FACE('',(#2410),#1468,.F.);
#16582=ADVANCED_FACE('',(#2411),#1469,.F.);
#16964=CLOSED_SHELL('',(#16523,#16524,#16525,#16526,#16527,#16528,#16529,
#16530,#16531,#16532,#16533,#16534,#16535,#16536,#16537,#16538,#16539,#16540,
#16541,#16542,#16543,#16544,#16545,#16546,#16547,#16548,#16549,#16550,#16551,
#16552,#16553,#16554,#16555,#16556,#16557,#16558,#16559,#16560,#16561,#16562,
#16563,#16564,#16565,#16566,#16567,#16568,#16569,#16570,#16571,#16572,#16573,
#16574,#16575,#16576,#16577,#16578,#16579,#16580,#16581,#16582));
#18218=AXIS2_PLACEMENT_3D('',#36456,#21369,#21370);
#18219=AXIS2_PLACEMENT_3D('',#36457,#21371,#21372);
#18220=AXIS2_PLACEMENT_3D('',#36459,#21373,#21374);
#18221=AXIS2_PLACEMENT_3D('',#36462,#21376,#21377);
#18222=AXIS2_PLACEMENT_3D('',#36463,#21378,#21379);
#18223=AXIS2_PLACEMENT_3D('',#36473,#21384,#21385);
#18224=AXIS2_PLACEMENT_3D('',#36475,#21386,#21387);
#18225=AXIS2_PLACEMENT_3D('',#36477,#21388,#21389);
#18226=AXIS2_PLACEMENT_3D('',#36479,#21390,#21391);
#18227=AXIS2_PLACEMENT_3D('',#36481,#21392,#21393);
#18228=AXIS2_PLACEMENT_3D('',#36482,#21394,#21395);
#18229=AXIS2_PLACEMENT_3D('',#36484,#21396,#21397);
#18230=AXIS2_PLACEMENT_3D('',#36486,#21399,#21400);
#18231=AXIS2_PLACEMENT_3D('',#36489,#21402,#21403);
#18232=AXIS2_PLACEMENT_3D('',#36490,#21404,#21405);
#18233=AXIS2_PLACEMENT_3D('',#36492,#21406,#21407);
#18234=AXIS2_PLACEMENT_3D('',#36494,#21409,#21410);
#18235=AXIS2_PLACEMENT_3D('',#36503,#21415,#21416);
#18236=AXIS2_PLACEMENT_3D('',#36505,#21417,#21418);
#18237=AXIS2_PLACEMENT_3D('',#36508,#21420,#21421);
#18238=AXIS2_PLACEMENT_3D('',#36509,#21422,#21423);
#18239=AXIS2_PLACEMENT_3D('',#36515,#21427,#21428);
#18240=AXIS2_PLACEMENT_3D('',#36517,#21429,#21430);
#18241=AXIS2_PLACEMENT_3D('',#36520,#21432,#21433);
#18242=AXIS2_PLACEMENT_3D('',#36521,#21434,#21435);
#18243=AXIS2_PLACEMENT_3D('',#36527,#21439,#21440);
#18244=AXIS2_PLACEMENT_3D('',#36529,#21441,#21442);
#18245=AXIS2_PLACEMENT_3D('',#36532,#21444,#21445);
#18246=AXIS2_PLACEMENT_3D('',#36533,#21446,#21447);
#18247=AXIS2_PLACEMENT_3D('',#36539,#21451,#21452);
#18248=AXIS2_PLACEMENT_3D('',#36540,#21453,#21454);
#18249=AXIS2_PLACEMENT_3D('',#36543,#21456,#21457);
#18250=AXIS2_PLACEMENT_3D('',#36544,#21458,#21459);
#18251=AXIS2_PLACEMENT_3D('',#36548,#21462,#21463);
#18252=AXIS2_PLACEMENT_3D('',#36550,#21464,#21465);
#18253=AXIS2_PLACEMENT_3D('',#36553,#21467,#21468);
#18254=AXIS2_PLACEMENT_3D('',#36554,#21469,#21470);
#18255=AXIS2_PLACEMENT_3D('',#36560,#21474,#21475);
#18256=AXIS2_PLACEMENT_3D('',#36562,#21476,#21477);
#18257=AXIS2_PLACEMENT_3D('',#36565,#21479,#21480);
#18258=AXIS2_PLACEMENT_3D('',#36566,#21481,#21482);
#18259=AXIS2_PLACEMENT_3D('',#36572,#21486,#21487);
#18260=AXIS2_PLACEMENT_3D('',#36574,#21488,#21489);
#18261=AXIS2_PLACEMENT_3D('',#36577,#21491,#21492);
#18262=AXIS2_PLACEMENT_3D('',#36578,#21493,#21494);
#18263=AXIS2_PLACEMENT_3D('',#36584,#21498,#21499);
#18264=AXIS2_PLACEMENT_3D('',#36585,#21500,#21501);
#18265=AXIS2_PLACEMENT_3D('',#36586,#21502,#21503);
#18266=AXIS2_PLACEMENT_3D('',#36587,#21504,#21505);
#18267=AXIS2_PLACEMENT_3D('',#36590,#21507,#21508);
#18268=AXIS2_PLACEMENT_3D('',#36591,#21509,#21510);
#18269=AXIS2_PLACEMENT_3D('',#36595,#21513,#21514);
#18270=AXIS2_PLACEMENT_3D('',#36598,#21516,#21517);
#18271=AXIS2_PLACEMENT_3D('',#36599,#21518,#21519);
#18272=AXIS2_PLACEMENT_3D('',#36603,#21522,#21523);
#18273=AXIS2_PLACEMENT_3D('',#36606,#21525,#21526);
#18274=AXIS2_PLACEMENT_3D('',#36607,#21527,#21528);
#18275=AXIS2_PLACEMENT_3D('',#36611,#21531,#21532);
#18276=AXIS2_PLACEMENT_3D('',#36614,#21534,#21535);
#18277=AXIS2_PLACEMENT_3D('',#36615,#21536,#21537);
#18278=AXIS2_PLACEMENT_3D('',#36620,#21540,#21541);
#18279=AXIS2_PLACEMENT_3D('',#36622,#21542,#21543);
#18280=AXIS2_PLACEMENT_3D('',#36624,#21544,#21545);
#18281=AXIS2_PLACEMENT_3D('',#36626,#21546,#21547);
#18282=AXIS2_PLACEMENT_3D('',#36628,#21548,#21549);
#18283=AXIS2_PLACEMENT_3D('',#36630,#21550,#21551);
#18284=AXIS2_PLACEMENT_3D('',#36631,#21552,#21553);
#18285=AXIS2_PLACEMENT_3D('',#36632,#21554,#21555);
#18286=AXIS2_PLACEMENT_3D('',#36638,#21559,#21560);
#18287=AXIS2_PLACEMENT_3D('',#36640,#21561,#21562);
#18288=AXIS2_PLACEMENT_3D('',#36643,#21564,#21565);
#18289=AXIS2_PLACEMENT_3D('',#36644,#21566,#21567);
#18290=AXIS2_PLACEMENT_3D('',#36650,#21571,#21572);
#18291=AXIS2_PLACEMENT_3D('',#36652,#21573,#21574);
#18292=AXIS2_PLACEMENT_3D('',#36655,#21576,#21577);
#18293=AXIS2_PLACEMENT_3D('',#36656,#21578,#21579);
#18294=AXIS2_PLACEMENT_3D('',#36662,#21583,#21584);
#18295=AXIS2_PLACEMENT_3D('',#36664,#21585,#21586);
#18296=AXIS2_PLACEMENT_3D('',#36667,#21588,#21589);
#18297=AXIS2_PLACEMENT_3D('',#36668,#21590,#21591);
#18298=AXIS2_PLACEMENT_3D('',#36674,#21595,#21596);
#18299=AXIS2_PLACEMENT_3D('',#36675,#21597,#21598);
#18300=AXIS2_PLACEMENT_3D('',#36678,#21600,#21601);
#18301=AXIS2_PLACEMENT_3D('',#36679,#21602,#21603);
#18302=AXIS2_PLACEMENT_3D('',#36683,#21606,#21607);
#18303=AXIS2_PLACEMENT_3D('',#36686,#21609,#21610);
#18304=AXIS2_PLACEMENT_3D('',#36687,#21611,#21612);
#18305=AXIS2_PLACEMENT_3D('',#36691,#21615,#21616);
#18306=AXIS2_PLACEMENT_3D('',#36694,#21618,#21619);
#18307=AXIS2_PLACEMENT_3D('',#36695,#21620,#21621);
#18308=AXIS2_PLACEMENT_3D('',#36699,#21624,#21625);
#18309=AXIS2_PLACEMENT_3D('',#36702,#21627,#21628);
#18310=AXIS2_PLACEMENT_3D('',#36703,#21629,#21630);
#18311=AXIS2_PLACEMENT_3D('',#36707,#21633,#21634);
#18312=AXIS2_PLACEMENT_3D('',#36708,#21635,#21636);
#18313=AXIS2_PLACEMENT_3D('',#36709,#21637,#21638);
#18314=AXIS2_PLACEMENT_3D('',#36711,#21640,#21641);
#18315=AXIS2_PLACEMENT_3D('',#36713,#21643,#21644);
#18316=AXIS2_PLACEMENT_3D('',#36715,#21646,#21647);
#18317=AXIS2_PLACEMENT_3D('',#36717,#21649,#21650);
#18318=AXIS2_PLACEMENT_3D('',#36719,#21652,#21653);
#18319=AXIS2_PLACEMENT_3D('',#36721,#21655,#21656);
#18320=AXIS2_PLACEMENT_3D('',#36722,#21657,#21658);
#18321=AXIS2_PLACEMENT_3D('',#36723,#21659,#21660);
#18322=AXIS2_PLACEMENT_3D('',#36725,#21662,#21663);
#18323=AXIS2_PLACEMENT_3D('',#36727,#21665,#21666);
#18324=AXIS2_PLACEMENT_3D('',#36729,#21668,#21669);
#18325=AXIS2_PLACEMENT_3D('',#36731,#21671,#21672);
#18326=AXIS2_PLACEMENT_3D('',#36733,#21674,#21675);
#21369=DIRECTION('axis',(0.,0.,1.));
#21370=DIRECTION('refdir',(1.,0.,0.));
#21371=DIRECTION('center_axis',(0.,0.,-1.));
#21372=DIRECTION('ref_axis',(1.,0.,0.));
#21373=DIRECTION('center_axis',(0.,0.,-1.));
#21374=DIRECTION('ref_axis',(1.,0.,0.));
#21375=DIRECTION('',(0.707106781186546,-8.65956056235491E-17,0.707106781186549));
#21376=DIRECTION('center_axis',(0.,0.,1.));
#21377=DIRECTION('ref_axis',(1.,0.,0.));
#21378=DIRECTION('center_axis',(0.,0.,-1.));
#21379=DIRECTION('ref_axis',(-1.,0.,0.));
#21380=DIRECTION('',(1.,0.,0.));
#21381=DIRECTION('',(0.,-1.,0.));
#21382=DIRECTION('',(-1.,0.,0.));
#21383=DIRECTION('',(0.,1.,0.));
#21384=DIRECTION('center_axis',(0.,0.,-1.));
#21385=DIRECTION('ref_axis',(1.,0.,0.));
#21386=DIRECTION('center_axis',(0.,0.,1.));
#21387=DIRECTION('ref_axis',(1.,0.,0.));
#21388=DIRECTION('center_axis',(0.,0.,1.));
#21389=DIRECTION('ref_axis',(1.,0.,0.));
#21390=DIRECTION('center_axis',(0.,0.,1.));
#21391=DIRECTION('ref_axis',(1.,0.,0.));
#21392=DIRECTION('center_axis',(0.,0.,1.));
#21393=DIRECTION('ref_axis',(1.,0.,0.));
#21394=DIRECTION('center_axis',(0.,0.,-1.));
#21395=DIRECTION('ref_axis',(1.,0.,0.));
#21396=DIRECTION('center_axis',(0.,0.,-1.));
#21397=DIRECTION('ref_axis',(1.,0.,0.));
#21398=DIRECTION('',(0.,0.,-1.));
#21399=DIRECTION('center_axis',(0.,0.,-1.));
#21400=DIRECTION('ref_axis',(1.,0.,0.));
#21401=DIRECTION('',(0.707106781186546,-8.65956056235491E-17,0.707106781186549));
#21402=DIRECTION('center_axis',(0.,0.,1.));
#21403=DIRECTION('ref_axis',(1.,0.,0.));
#21404=DIRECTION('center_axis',(0.,0.,-1.));
#21405=DIRECTION('ref_axis',(1.,0.,0.));
#21406=DIRECTION('center_axis',(0.,0.,-1.));
#21407=DIRECTION('ref_axis',(1.,0.,0.));
#21408=DIRECTION('',(0.,0.,-1.));
#21409=DIRECTION('center_axis',(0.,-0.707106781186541,0.707106781186554));
#21410=DIRECTION('ref_axis',(1.,0.,0.));
#21411=DIRECTION('',(0.,-0.707106781186554,-0.707106781186541));
#21412=DIRECTION('',(1.,0.,0.));
#21413=DIRECTION('',(0.,0.707106781186554,0.707106781186541));
#21414=DIRECTION('',(-1.,0.,0.));
#21415=DIRECTION('center_axis',(0.,1.,0.));
#21416=DIRECTION('ref_axis',(-0.707106781186548,0.,0.707106781186548));
#21417=DIRECTION('center_axis',(0.,-1.,0.));
#21418=DIRECTION('ref_axis',(-0.707106781186548,0.,0.707106781186548));
#21419=DIRECTION('',(0.707106781186551,-0.707106781186544,0.));
#21420=DIRECTION('center_axis',(0.,1.,0.));
#21421=DIRECTION('ref_axis',(-0.707106781186547,0.,0.707106781186547));
#21422=DIRECTION('center_axis',(-0.707106781186554,-0.707106781186541,0.));
#21423=DIRECTION('ref_axis',(0.,0.,1.));
#21424=DIRECTION('',(0.707106781186541,-0.707106781186554,0.));
#21425=DIRECTION('',(0.,0.,1.));
#21426=DIRECTION('',(0.,0.,-1.));
#21427=DIRECTION('center_axis',(0.,1.,0.));
#21428=DIRECTION('ref_axis',(-0.707106781186548,0.,-0.707106781186548));
#21429=DIRECTION('center_axis',(0.,-1.,0.));
#21430=DIRECTION('ref_axis',(-0.707106781186548,0.,-0.707106781186548));
#21431=DIRECTION('',(0.,-0.707106781186547,0.707106781186548));
#21432=DIRECTION('center_axis',(0.,1.,0.));
#21433=DIRECTION('ref_axis',(-0.707106781186547,0.,-0.707106781186547));
#21434=DIRECTION('center_axis',(0.,-0.707106781186543,-0.707106781186552));
#21435=DIRECTION('ref_axis',(-1.,0.,0.));
#21436=DIRECTION('',(0.,-0.707106781186552,0.707106781186543));
#21437=DIRECTION('',(-1.,0.,0.));
#21438=DIRECTION('',(1.,0.,0.));
#21439=DIRECTION('center_axis',(0.,1.,0.));
#21440=DIRECTION('ref_axis',(0.707106781186548,0.,-0.707106781186548));
#21441=DIRECTION('center_axis',(0.,-1.,0.));
#21442=DIRECTION('ref_axis',(0.707106781186548,0.,-0.707106781186548));
#21443=DIRECTION('',(-0.707106781186554,-0.707106781186541,0.));
#21444=DIRECTION('center_axis',(0.,1.,0.));
#21445=DIRECTION('ref_axis',(0.707106781186547,0.,-0.707106781186547));
#21446=DIRECTION('center_axis',(0.707106781186554,-0.707106781186541,0.));
#21447=DIRECTION('ref_axis',(0.,0.,-1.));
#21448=DIRECTION('',(-0.707106781186541,-0.707106781186554,0.));
#21449=DIRECTION('',(0.,0.,-1.));
#21450=DIRECTION('',(0.,0.,1.));
#21451=DIRECTION('center_axis',(0.,-1.,0.));
#21452=DIRECTION('ref_axis',(-0.707106781186548,0.,0.707106781186548));
#21453=DIRECTION('center_axis',(0.,1.,0.));
#21454=DIRECTION('ref_axis',(-0.707106781186548,0.,0.707106781186548));
#21455=DIRECTION('',(0.,-0.707106781186546,0.707106781186549));
#21456=DIRECTION('center_axis',(0.,-1.,0.));
#21457=DIRECTION('ref_axis',(-0.707106781186547,0.,0.707106781186547));
#21458=DIRECTION('center_axis',(0.,-0.707106781186543,-0.707106781186552));
#21459=DIRECTION('ref_axis',(-1.,0.,0.));
#21460=DIRECTION('',(0.,-0.707106781186552,0.707106781186543));
#21461=DIRECTION('',(-1.,0.,0.));
#21462=DIRECTION('center_axis',(0.,-1.,0.));
#21463=DIRECTION('ref_axis',(0.707106781186548,0.,0.707106781186548));
#21464=DIRECTION('center_axis',(0.,1.,0.));
#21465=DIRECTION('ref_axis',(0.707106781186548,0.,0.707106781186548));
#21466=DIRECTION('',(0.707106781186554,-0.707106781186541,0.));
#21467=DIRECTION('center_axis',(0.,-1.,0.));
#21468=DIRECTION('ref_axis',(0.707106781186547,0.,0.707106781186547));
#21469=DIRECTION('center_axis',(-0.707106781186548,-0.707106781186548,0.));
#21470=DIRECTION('ref_axis',(0.,0.,1.));
#21471=DIRECTION('',(0.707106781186547,-0.707106781186547,0.));
#21472=DIRECTION('',(0.,0.,1.));
#21473=DIRECTION('',(0.,0.,-1.));
#21474=DIRECTION('center_axis',(0.,1.,0.));
#21475=DIRECTION('ref_axis',(-0.707106781186555,0.,-0.70710678118654));
#21476=DIRECTION('center_axis',(0.,-1.,0.));
#21477=DIRECTION('ref_axis',(-0.707106781186555,0.,-0.70710678118654));
#21478=DIRECTION('',(0.,-0.707106781186547,0.707106781186548));
#21479=DIRECTION('center_axis',(0.,1.,0.));
#21480=DIRECTION('ref_axis',(-0.707106781186555,0.,-0.70710678118654));
#21481=DIRECTION('center_axis',(0.,-0.707106781186543,-0.707106781186552));
#21482=DIRECTION('ref_axis',(-1.,0.,0.));
#21483=DIRECTION('',(0.,-0.707106781186552,0.707106781186543));
#21484=DIRECTION('',(-1.,0.,0.));
#21485=DIRECTION('',(1.,0.,0.));
#21486=DIRECTION('center_axis',(0.,1.,0.));
#21487=DIRECTION('ref_axis',(0.70710678118654,0.,-0.707106781186555));
#21488=DIRECTION('center_axis',(0.,-1.,0.));
#21489=DIRECTION('ref_axis',(0.70710678118654,0.,-0.707106781186555));
#21490=DIRECTION('',(-0.707106781186529,-0.707106781186566,0.));
#21491=DIRECTION('center_axis',(0.,1.,0.));
#21492=DIRECTION('ref_axis',(0.70710678118654,0.,-0.707106781186555));
#21493=DIRECTION('center_axis',(0.707106781186548,-0.707106781186548,0.));
#21494=DIRECTION('ref_axis',(0.,0.,-1.));
#21495=DIRECTION('',(-0.707106781186547,-0.707106781186547,0.));
#21496=DIRECTION('',(0.,0.,-1.));
#21497=DIRECTION('',(0.,0.,1.));
#21498=DIRECTION('center_axis',(0.,1.,0.));
#21499=DIRECTION('ref_axis',(0.707106781186555,0.,0.70710678118654));
#21500=DIRECTION('center_axis',(0.,-1.,0.));
#21501=DIRECTION('ref_axis',(0.707106781186555,0.,0.70710678118654));
#21502=DIRECTION('center_axis',(0.,1.,0.));
#21503=DIRECTION('ref_axis',(0.707106781186555,0.,0.70710678118654));
#21504=DIRECTION('center_axis',(0.,1.,0.));
#21505=DIRECTION('ref_axis',(-0.707106781186548,0.,0.707106781186548));
#21506=DIRECTION('',(0.,1.,0.));
#21507=DIRECTION('center_axis',(0.,-1.,0.));
#21508=DIRECTION('ref_axis',(-0.707106781186548,0.,0.707106781186548));
#21509=DIRECTION('center_axis',(1.,0.,0.));
#21510=DIRECTION('ref_axis',(0.,0.,-1.));
#21511=DIRECTION('',(0.,-1.,0.));
#21512=DIRECTION('',(0.,0.,-1.));
#21513=DIRECTION('center_axis',(0.,1.,0.));
#21514=DIRECTION('ref_axis',(0.707106781186548,0.,-0.707106781186548));
#21515=DIRECTION('',(0.,1.,0.));
#21516=DIRECTION('center_axis',(0.,1.,0.));
#21517=DIRECTION('ref_axis',(0.707106781186548,0.,-0.707106781186548));
#21518=DIRECTION('center_axis',(0.,0.,-1.));
#21519=DIRECTION('ref_axis',(-1.,0.,0.));
#21520=DIRECTION('',(0.,-1.,0.));
#21521=DIRECTION('',(-1.,0.,0.));
#21522=DIRECTION('center_axis',(0.,1.,0.));
#21523=DIRECTION('ref_axis',(-0.707106781186548,0.,-0.707106781186548));
#21524=DIRECTION('',(0.,1.,0.));
#21525=DIRECTION('center_axis',(0.,1.,0.));
#21526=DIRECTION('ref_axis',(-0.707106781186548,0.,-0.707106781186548));
#21527=DIRECTION('center_axis',(-1.,0.,0.));
#21528=DIRECTION('ref_axis',(0.,0.,1.));
#21529=DIRECTION('',(0.,-1.,0.));
#21530=DIRECTION('',(0.,0.,1.));
#21531=DIRECTION('center_axis',(0.,1.,0.));
#21532=DIRECTION('ref_axis',(-0.707106781186548,0.,0.707106781186548));
#21533=DIRECTION('',(0.,1.,0.));
#21534=DIRECTION('center_axis',(0.,1.,0.));
#21535=DIRECTION('ref_axis',(-0.707106781186548,0.,0.707106781186548));
#21536=DIRECTION('center_axis',(0.,0.,1.));
#21537=DIRECTION('ref_axis',(1.,0.,0.));
#21538=DIRECTION('',(0.,-1.,0.));
#21539=DIRECTION('',(1.,0.,0.));
#21540=DIRECTION('center_axis',(0.,0.,1.));
#21541=DIRECTION('ref_axis',(1.,0.,0.));
#21542=DIRECTION('center_axis',(0.,0.,-1.));
#21543=DIRECTION('ref_axis',(1.,0.,0.));
#21544=DIRECTION('center_axis',(0.,0.,-1.));
#21545=DIRECTION('ref_axis',(1.,0.,0.));
#21546=DIRECTION('center_axis',(0.,0.,-1.));
#21547=DIRECTION('ref_axis',(1.,0.,0.));
#21548=DIRECTION('center_axis',(0.,0.,-1.));
#21549=DIRECTION('ref_axis',(1.,0.,0.));
#21550=DIRECTION('center_axis',(0.,0.,1.));
#21551=DIRECTION('ref_axis',(1.,0.,0.));
#21552=DIRECTION('center_axis',(0.,1.,0.));
#21553=DIRECTION('ref_axis',(1.,0.,0.));
#21554=DIRECTION('center_axis',(0.,0.707106781186541,0.707106781186554));
#21555=DIRECTION('ref_axis',(1.,0.,0.));
#21556=DIRECTION('',(0.,0.707106781186554,-0.707106781186541));
#21557=DIRECTION('',(-1.,0.,0.));
#21558=DIRECTION('',(0.,-0.707106781186554,0.707106781186541));
#21559=DIRECTION('center_axis',(0.,-1.,0.));
#21560=DIRECTION('ref_axis',(0.707106781186555,0.,0.70710678118654));
#21561=DIRECTION('center_axis',(0.,1.,0.));
#21562=DIRECTION('ref_axis',(0.707106781186555,0.,0.70710678118654));
#21563=DIRECTION('',(-0.707106781186535,0.70710678118656,0.));
#21564=DIRECTION('center_axis',(0.,-1.,0.));
#21565=DIRECTION('ref_axis',(0.707106781186555,0.,0.70710678118654));
#21566=DIRECTION('center_axis',(0.707106781186548,0.707106781186548,0.));
#21567=DIRECTION('ref_axis',(0.,0.,-1.));
#21568=DIRECTION('',(-0.707106781186547,0.707106781186547,0.));
#21569=DIRECTION('',(0.,0.,1.));
#21570=DIRECTION('',(0.,0.,-1.));
#21571=DIRECTION('center_axis',(0.,-1.,0.));
#21572=DIRECTION('ref_axis',(0.70710678118654,0.,-0.707106781186555));
#21573=DIRECTION('center_axis',(0.,1.,0.));
#21574=DIRECTION('ref_axis',(0.70710678118654,0.,-0.707106781186555));
#21575=DIRECTION('',(0.,0.707106781186553,0.707106781186542));
#21576=DIRECTION('center_axis',(0.,-1.,0.));
#21577=DIRECTION('ref_axis',(0.70710678118654,0.,-0.707106781186555));
#21578=DIRECTION('center_axis',(0.,0.707106781186543,-0.707106781186552));
#21579=DIRECTION('ref_axis',(-1.,0.,0.));
#21580=DIRECTION('',(0.,0.707106781186552,0.707106781186543));
#21581=DIRECTION('',(1.,0.,0.));
#21582=DIRECTION('',(-1.,0.,0.));
#21583=DIRECTION('center_axis',(0.,-1.,0.));
#21584=DIRECTION('ref_axis',(-0.707106781186555,0.,-0.70710678118654));
#21585=DIRECTION('center_axis',(0.,1.,0.));
#21586=DIRECTION('ref_axis',(-0.707106781186555,0.,-0.70710678118654));
#21587=DIRECTION('',(0.707106781186535,0.70710678118656,0.));
#21588=DIRECTION('center_axis',(0.,-1.,0.));
#21589=DIRECTION('ref_axis',(-0.707106781186555,0.,-0.70710678118654));
#21590=DIRECTION('center_axis',(-0.707106781186548,0.707106781186548,0.));
#21591=DIRECTION('ref_axis',(0.,0.,1.));
#21592=DIRECTION('',(0.707106781186547,0.707106781186547,0.));
#21593=DIRECTION('',(0.,0.,-1.));
#21594=DIRECTION('',(0.,0.,1.));
#21595=DIRECTION('center_axis',(0.,1.,0.));
#21596=DIRECTION('ref_axis',(0.707106781186548,0.,0.707106781186548));
#21597=DIRECTION('center_axis',(0.,-1.,0.));
#21598=DIRECTION('ref_axis',(0.707106781186548,0.,0.707106781186548));
#21599=DIRECTION('',(0.,0.707106781186554,0.707106781186541));
#21600=DIRECTION('center_axis',(0.,1.,0.));
#21601=DIRECTION('ref_axis',(0.707106781186547,0.,0.707106781186547));
#21602=DIRECTION('center_axis',(0.,0.707106781186543,-0.707106781186552));
#21603=DIRECTION('ref_axis',(-1.,0.,0.));
#21604=DIRECTION('',(0.,0.707106781186552,0.707106781186543));
#21605=DIRECTION('',(1.,0.,0.));
#21606=DIRECTION('center_axis',(0.,1.,0.));
#21607=DIRECTION('ref_axis',(-0.707106781186548,0.,0.707106781186548));
#21608=DIRECTION('',(-0.707106781186547,0.707106781186547,0.));
#21609=DIRECTION('center_axis',(0.,1.,0.));
#21610=DIRECTION('ref_axis',(-0.707106781186547,0.,0.707106781186547));
#21611=DIRECTION('center_axis',(0.707106781186554,0.707106781186541,0.));
#21612=DIRECTION('ref_axis',(0.,0.,-1.));
#21613=DIRECTION('',(-0.707106781186541,0.707106781186554,0.));
#21614=DIRECTION('',(0.,0.,1.));
#21615=DIRECTION('center_axis',(0.,-1.,0.));
#21616=DIRECTION('ref_axis',(0.707106781186548,0.,-0.707106781186548));
#21617=DIRECTION('',(0.,0.707106781186553,0.707106781186542));
#21618=DIRECTION('center_axis',(0.,-1.,0.));
#21619=DIRECTION('ref_axis',(0.707106781186547,0.,-0.707106781186547));
#21620=DIRECTION('center_axis',(0.,0.707106781186543,-0.707106781186552));
#21621=DIRECTION('ref_axis',(-1.,0.,0.));
#21622=DIRECTION('',(0.,0.707106781186552,0.707106781186543));
#21623=DIRECTION('',(1.,0.,0.));
#21624=DIRECTION('center_axis',(0.,-1.,0.));
#21625=DIRECTION('ref_axis',(-0.707106781186548,0.,-0.707106781186548));
#21626=DIRECTION('',(0.707106781186541,0.707106781186554,0.));
#21627=DIRECTION('center_axis',(0.,-1.,0.));
#21628=DIRECTION('ref_axis',(-0.707106781186547,0.,-0.707106781186547));
#21629=DIRECTION('center_axis',(-0.707106781186554,0.707106781186541,0.));
#21630=DIRECTION('ref_axis',(0.,0.,1.));
#21631=DIRECTION('',(0.707106781186541,0.707106781186554,0.));
#21632=DIRECTION('',(0.,0.,-1.));
#21633=DIRECTION('center_axis',(0.,-1.,0.));
#21634=DIRECTION('ref_axis',(-0.707106781186548,0.,0.707106781186548));
#21635=DIRECTION('center_axis',(0.,-1.,0.));
#21636=DIRECTION('ref_axis',(-0.707106781186547,0.,0.707106781186547));
#21637=DIRECTION('center_axis',(0.,1.,0.));
#21638=DIRECTION('ref_axis',(0.707106781186548,0.,0.707106781186548));
#21639=DIRECTION('',(0.,-1.,0.));
#21640=DIRECTION('center_axis',(-1.,0.,0.));
#21641=DIRECTION('ref_axis',(0.,0.,1.));
#21642=DIRECTION('',(0.,1.,0.));
#21643=DIRECTION('center_axis',(0.,1.,0.));
#21644=DIRECTION('ref_axis',(-0.707106781186555,0.,-0.70710678118654));
#21645=DIRECTION('',(0.,-1.,0.));
#21646=DIRECTION('center_axis',(0.,0.,-1.));
#21647=DIRECTION('ref_axis',(-1.,0.,0.));
#21648=DIRECTION('',(0.,1.,0.));
#21649=DIRECTION('center_axis',(0.,1.,0.));
#21650=DIRECTION('ref_axis',(0.70710678118654,0.,-0.707106781186555));
#21651=DIRECTION('',(0.,-1.,0.));
#21652=DIRECTION('center_axis',(1.,0.,0.));
#21653=DIRECTION('ref_axis',(0.,0.,-1.));
#21654=DIRECTION('',(0.,1.,0.));
#21655=DIRECTION('center_axis',(0.,1.,0.));
#21656=DIRECTION('ref_axis',(0.707106781186555,0.,0.70710678118654));
#21657=DIRECTION('center_axis',(0.,1.,0.));
#21658=DIRECTION('ref_axis',(0.,0.,1.));
#21659=DIRECTION('center_axis',(0.,0.,1.));
#21660=DIRECTION('ref_axis',(1.,0.,0.));
#21661=DIRECTION('',(0.707106781186548,8.65956056235493E-17,-0.707106781186548));
#21662=DIRECTION('center_axis',(0.,0.,1.));
#21663=DIRECTION('ref_axis',(1.,0.,0.));
#21664=DIRECTION('',(0.707106781186548,8.65956056235493E-17,-0.707106781186548));
#21665=DIRECTION('center_axis',(0.,0.,-1.));
#21666=DIRECTION('ref_axis',(1.,0.,0.));
#21667=DIRECTION('',(0.,0.,-1.));
#21668=DIRECTION('center_axis',(0.,0.,-1.));
#21669=DIRECTION('ref_axis',(1.,0.,0.));
#21670=DIRECTION('',(0.,0.,-1.));
#21671=DIRECTION('center_axis',(0.,0.,-1.));
#21672=DIRECTION('ref_axis',(1.,0.,0.));
#21673=DIRECTION('',(0.,0.,-1.));
#21674=DIRECTION('center_axis',(0.,0.,-1.));
#21675=DIRECTION('ref_axis',(1.,0.,0.));
#21676=DIRECTION('',(0.,0.,-1.));
#36456=CARTESIAN_POINT('',(0.,0.,0.));
#36457=CARTESIAN_POINT('Origin',(61.,-66.,18.25));
#36458=CARTESIAN_POINT('',(57.,-66.,18.));
#36459=CARTESIAN_POINT('Origin',(61.,-66.,18.));
#36460=CARTESIAN_POINT('',(57.5,-66.,18.5));
#36461=CARTESIAN_POINT('',(57.25,-66.,18.25));
#36462=CARTESIAN_POINT('Origin',(61.,-66.,18.5));
#36463=CARTESIAN_POINT('Origin',(80.,-72.5,18.));
#36464=CARTESIAN_POINT('',(42.8,-72.,18.));
#36465=CARTESIAN_POINT('',(79.2,-72.,18.));
#36466=CARTESIAN_POINT('',(70.5,-72.,18.));
#36467=CARTESIAN_POINT('',(42.8,72.,18.));
#36468=CARTESIAN_POINT('',(42.8,-72.5,18.));
#36469=CARTESIAN_POINT('',(79.2,72.,18.));
#36470=CARTESIAN_POINT('',(70.5,72.,18.));
#36471=CARTESIAN_POINT('',(79.2,-72.5,18.));
#36472=CARTESIAN_POINT('',(57.,66.,18.));
#36473=CARTESIAN_POINT('Origin',(61.,66.,18.));
#36474=CARTESIAN_POINT('',(56.5,52.5,18.));
#36475=CARTESIAN_POINT('Origin',(61.,52.5,18.));
#36476=CARTESIAN_POINT('',(56.5,-25.,18.));
#36477=CARTESIAN_POINT('Origin',(61.,-25.,18.));
#36478=CARTESIAN_POINT('',(56.5,25.,18.));
#36479=CARTESIAN_POINT('Origin',(61.,25.,18.));
#36480=CARTESIAN_POINT('',(56.5,-52.5,18.));
#36481=CARTESIAN_POINT('Origin',(61.,-52.5,18.));
#36482=CARTESIAN_POINT('Origin',(61.,-66.,21.));
#36483=CARTESIAN_POINT('',(57.5,-66.,20.5));
#36484=CARTESIAN_POINT('Origin',(61.,-66.,20.5));
#36485=CARTESIAN_POINT('',(57.5,-66.,21.));
#36486=CARTESIAN_POINT('Origin',(61.,66.,18.25));
#36487=CARTESIAN_POINT('',(57.5,66.,18.5));
#36488=CARTESIAN_POINT('',(57.25,66.,18.25));
#36489=CARTESIAN_POINT('Origin',(61.,66.,18.5));
#36490=CARTESIAN_POINT('Origin',(61.,66.,21.));
#36491=CARTESIAN_POINT('',(57.5,66.,20.5));
#36492=CARTESIAN_POINT('Origin',(61.,66.,20.5));
#36493=CARTESIAN_POINT('',(57.5,66.,21.));
#36494=CARTESIAN_POINT('Origin',(50.,-72.25,20.75));
#36495=CARTESIAN_POINT('',(39.8,-72.,21.));
#36496=CARTESIAN_POINT('',(39.8,-72.5,20.5));
#36497=CARTESIAN_POINT('',(39.8,-72.,21.));
#36498=CARTESIAN_POINT('',(82.2,-72.5,20.5));
#36499=CARTESIAN_POINT('',(50.,-72.5,20.5));
#36500=CARTESIAN_POINT('',(82.2,-72.,21.));
#36501=CARTESIAN_POINT('',(82.2,-72.5,20.5));
#36502=CARTESIAN_POINT('',(50.,-72.,21.));
#36503=CARTESIAN_POINT('Origin',(39.8,-72.25,20.2));
#36504=CARTESIAN_POINT('',(39.,-72.,20.2));
#36505=CARTESIAN_POINT('Origin',(39.8,-72.,20.2));
#36506=CARTESIAN_POINT('',(39.5,-72.5,20.2));
#36507=CARTESIAN_POINT('',(39.,-72.,20.2));
#36508=CARTESIAN_POINT('Origin',(39.8,-72.5,20.2));
#36509=CARTESIAN_POINT('Origin',(39.25,-72.25,9.75));
#36510=CARTESIAN_POINT('',(39.,-72.,6.8));
#36511=CARTESIAN_POINT('',(39.5,-72.5,6.8));
#36512=CARTESIAN_POINT('',(39.,-72.,6.8));
#36513=CARTESIAN_POINT('',(39.5,-72.5,9.75));
#36514=CARTESIAN_POINT('',(39.,-72.,9.75));
#36515=CARTESIAN_POINT('Origin',(39.8,-72.25,6.8));
#36516=CARTESIAN_POINT('',(39.8,-72.,6.));
#36517=CARTESIAN_POINT('Origin',(39.8,-72.,6.8));
#36518=CARTESIAN_POINT('',(39.8,-72.5,6.5));
#36519=CARTESIAN_POINT('',(39.8,-72.,6.));
#36520=CARTESIAN_POINT('Origin',(39.8,-72.5,6.8));
#36521=CARTESIAN_POINT('Origin',(51.5,-72.25,6.25));
#36522=CARTESIAN_POINT('',(41.2,-72.,6.));
#36523=CARTESIAN_POINT('',(41.2,-72.5,6.5));
#36524=CARTESIAN_POINT('',(41.2,-72.,6.));
#36525=CARTESIAN_POINT('',(51.5,-72.5,6.5));
#36526=CARTESIAN_POINT('',(51.5,-72.,6.));
#36527=CARTESIAN_POINT('Origin',(41.2,-72.25,6.8));
#36528=CARTESIAN_POINT('',(42.,-72.,6.8));
#36529=CARTESIAN_POINT('Origin',(41.2,-72.,6.8));
#36530=CARTESIAN_POINT('',(41.5,-72.5,6.8));
#36531=CARTESIAN_POINT('',(42.,-72.,6.8));
#36532=CARTESIAN_POINT('Origin',(41.2,-72.5,6.8));
#36533=CARTESIAN_POINT('Origin',(41.75,-72.25,15.75));
#36534=CARTESIAN_POINT('',(42.,-72.,17.2));
#36535=CARTESIAN_POINT('',(41.5,-72.5,17.2));
#36536=CARTESIAN_POINT('',(42.,-72.,17.2));
#36537=CARTESIAN_POINT('',(41.5,-72.5,15.75));
#36538=CARTESIAN_POINT('',(42.,-72.,15.75));
#36539=CARTESIAN_POINT('Origin',(42.8,-72.25,17.2));
#36540=CARTESIAN_POINT('Origin',(42.8,-72.,17.2));
#36541=CARTESIAN_POINT('',(42.8,-72.5,18.5));
#36542=CARTESIAN_POINT('',(42.8,-72.,18.));
#36543=CARTESIAN_POINT('Origin',(42.8,-72.5,17.2));
#36544=CARTESIAN_POINT('Origin',(70.5,-72.25,18.25));
#36545=CARTESIAN_POINT('',(79.2,-72.5,18.5));
#36546=CARTESIAN_POINT('',(79.2,-72.,18.));
#36547=CARTESIAN_POINT('',(70.5,-72.5,18.5));
#36548=CARTESIAN_POINT('Origin',(79.2,-72.25,17.2));
#36549=CARTESIAN_POINT('',(80.,-72.,17.2));
#36550=CARTESIAN_POINT('Origin',(79.2,-72.,17.2));
#36551=CARTESIAN_POINT('',(80.5,-72.5,17.2));
#36552=CARTESIAN_POINT('',(80.,-72.,17.2));
#36553=CARTESIAN_POINT('Origin',(79.2,-72.5,17.2));
#36554=CARTESIAN_POINT('Origin',(80.25,-72.25,9.75));
#36555=CARTESIAN_POINT('',(80.,-72.,6.8));
#36556=CARTESIAN_POINT('',(80.5,-72.5,6.8));
#36557=CARTESIAN_POINT('',(80.,-72.,6.8));
#36558=CARTESIAN_POINT('',(80.5,-72.5,9.75));
#36559=CARTESIAN_POINT('',(80.,-72.,9.75));
#36560=CARTESIAN_POINT('Origin',(80.8,-72.25,6.8));
#36561=CARTESIAN_POINT('',(80.8,-72.,6.));
#36562=CARTESIAN_POINT('Origin',(80.8,-72.,6.8));
#36563=CARTESIAN_POINT('',(80.8,-72.5,6.5));
#36564=CARTESIAN_POINT('',(80.8,-72.,6.));
#36565=CARTESIAN_POINT('Origin',(80.8,-72.5,6.8));
#36566=CARTESIAN_POINT('Origin',(72.,-72.25,6.25));
#36567=CARTESIAN_POINT('',(82.2,-72.,6.));
#36568=CARTESIAN_POINT('',(82.2,-72.5,6.5));
#36569=CARTESIAN_POINT('',(82.2,-72.,6.));
#36570=CARTESIAN_POINT('',(72.,-72.5,6.5));
#36571=CARTESIAN_POINT('',(72.,-72.,6.));
#36572=CARTESIAN_POINT('Origin',(82.2,-72.25,6.8));
#36573=CARTESIAN_POINT('',(83.,-72.,6.8));
#36574=CARTESIAN_POINT('Origin',(82.2,-72.,6.8));
#36575=CARTESIAN_POINT('',(82.5,-72.5,6.8));
#36576=CARTESIAN_POINT('',(83.,-72.,6.8));
#36577=CARTESIAN_POINT('Origin',(82.2,-72.5,6.8));
#36578=CARTESIAN_POINT('Origin',(82.75,-72.25,17.25));
#36579=CARTESIAN_POINT('',(83.,-72.,20.2));
#36580=CARTESIAN_POINT('',(82.5,-72.5,20.2));
#36581=CARTESIAN_POINT('',(83.,-72.,20.2));
#36582=CARTESIAN_POINT('',(82.5,-72.5,17.25));
#36583=CARTESIAN_POINT('',(83.,-72.,17.25));
#36584=CARTESIAN_POINT('Origin',(82.2,-72.25,20.2));
#36585=CARTESIAN_POINT('Origin',(82.2,-72.,20.2));
#36586=CARTESIAN_POINT('Origin',(82.2,-72.5,20.2));
#36587=CARTESIAN_POINT('Origin',(42.8,-72.5,17.2));
#36588=CARTESIAN_POINT('',(42.,72.,17.2));
#36589=CARTESIAN_POINT('',(42.,-72.5,17.2));
#36590=CARTESIAN_POINT('Origin',(42.8,72.,17.2));
#36591=CARTESIAN_POINT('Origin',(42.,-72.5,18.));
#36592=CARTESIAN_POINT('',(42.,72.,6.8));
#36593=CARTESIAN_POINT('',(42.,-72.5,6.8));
#36594=CARTESIAN_POINT('',(42.,72.,15.75));
#36595=CARTESIAN_POINT('Origin',(41.2,-72.5,6.8));
#36596=CARTESIAN_POINT('',(41.2,72.,6.));
#36597=CARTESIAN_POINT('',(41.2,-72.5,6.));
#36598=CARTESIAN_POINT('Origin',(41.2,72.,6.8));
#36599=CARTESIAN_POINT('Origin',(42.,-72.5,6.));
#36600=CARTESIAN_POINT('',(39.8,72.,6.));
#36601=CARTESIAN_POINT('',(39.8,-72.5,6.));
#36602=CARTESIAN_POINT('',(51.5,72.,6.));
#36603=CARTESIAN_POINT('Origin',(39.8,-72.5,6.8));
#36604=CARTESIAN_POINT('',(39.,72.,6.8));
#36605=CARTESIAN_POINT('',(39.,-72.5,6.8));
#36606=CARTESIAN_POINT('Origin',(39.8,72.,6.8));
#36607=CARTESIAN_POINT('Origin',(39.,-72.5,6.));
#36608=CARTESIAN_POINT('',(39.,72.,20.2));
#36609=CARTESIAN_POINT('',(39.,-72.5,20.2));
#36610=CARTESIAN_POINT('',(39.,72.,9.75));
#36611=CARTESIAN_POINT('Origin',(39.8,-72.5,20.2));
#36612=CARTESIAN_POINT('',(39.8,72.,21.));
#36613=CARTESIAN_POINT('',(39.8,-72.5,21.));
#36614=CARTESIAN_POINT('Origin',(39.8,72.,20.2));
#36615=CARTESIAN_POINT('Origin',(39.,-72.5,21.));
#36616=CARTESIAN_POINT('',(82.2,72.,21.));
#36617=CARTESIAN_POINT('',(82.2,-72.5,21.));
#36618=CARTESIAN_POINT('',(50.,72.,21.));
#36619=CARTESIAN_POINT('',(57.,-66.,21.));
#36620=CARTESIAN_POINT('Origin',(61.,-66.,21.));
#36621=CARTESIAN_POINT('',(56.5,-52.5,21.));
#36622=CARTESIAN_POINT('Origin',(61.,-52.5,21.));
#36623=CARTESIAN_POINT('',(56.5,25.,21.));
#36624=CARTESIAN_POINT('Origin',(61.,25.,21.));
#36625=CARTESIAN_POINT('',(56.5,-25.,21.));
#36626=CARTESIAN_POINT('Origin',(61.,-25.,21.));
#36627=CARTESIAN_POINT('',(56.5,52.5,21.));
#36628=CARTESIAN_POINT('Origin',(61.,52.5,21.));
#36629=CARTESIAN_POINT('',(57.,66.,21.));
#36630=CARTESIAN_POINT('Origin',(61.,66.,21.));
#36631=CARTESIAN_POINT('Origin',(61.,-72.5,13.5));
#36632=CARTESIAN_POINT('Origin',(50.,72.25,20.75));
#36633=CARTESIAN_POINT('',(82.2,72.5,20.5));
#36634=CARTESIAN_POINT('',(82.2,72.,21.));
#36635=CARTESIAN_POINT('',(39.8,72.5,20.5));
#36636=CARTESIAN_POINT('',(50.,72.5,20.5));
#36637=CARTESIAN_POINT('',(39.8,72.5,20.5));
#36638=CARTESIAN_POINT('Origin',(82.2,72.25,20.2));
#36639=CARTESIAN_POINT('',(83.,72.,20.2));
#36640=CARTESIAN_POINT('Origin',(82.2,72.,20.2));
#36641=CARTESIAN_POINT('',(82.5,72.5,20.2));
#36642=CARTESIAN_POINT('',(83.,72.,20.2));
#36643=CARTESIAN_POINT('Origin',(82.2,72.5,20.2));
#36644=CARTESIAN_POINT('Origin',(82.75,72.25,17.25));
#36645=CARTESIAN_POINT('',(83.,72.,6.8));
#36646=CARTESIAN_POINT('',(82.5,72.5,6.8));
#36647=CARTESIAN_POINT('',(83.,72.,6.8));
#36648=CARTESIAN_POINT('',(82.5,72.5,17.25));
#36649=CARTESIAN_POINT('',(83.,72.,17.25));
#36650=CARTESIAN_POINT('Origin',(82.2,72.25,6.8));
#36651=CARTESIAN_POINT('',(82.2,72.,6.));
#36652=CARTESIAN_POINT('Origin',(82.2,72.,6.8));
#36653=CARTESIAN_POINT('',(82.2,72.5,6.5));
#36654=CARTESIAN_POINT('',(82.2,72.,6.));
#36655=CARTESIAN_POINT('Origin',(82.2,72.5,6.8));
#36656=CARTESIAN_POINT('Origin',(72.,72.25,6.25));
#36657=CARTESIAN_POINT('',(80.8,72.,6.));
#36658=CARTESIAN_POINT('',(80.8,72.5,6.5));
#36659=CARTESIAN_POINT('',(80.8,72.,6.));
#36660=CARTESIAN_POINT('',(72.,72.5,6.5));
#36661=CARTESIAN_POINT('',(72.,72.,6.));
#36662=CARTESIAN_POINT('Origin',(80.8,72.25,6.8));
#36663=CARTESIAN_POINT('',(80.,72.,6.8));
#36664=CARTESIAN_POINT('Origin',(80.8,72.,6.8));
#36665=CARTESIAN_POINT('',(80.5,72.5,6.8));
#36666=CARTESIAN_POINT('',(80.,72.,6.8));
#36667=CARTESIAN_POINT('Origin',(80.8,72.5,6.8));
#36668=CARTESIAN_POINT('Origin',(80.25,72.25,9.75));
#36669=CARTESIAN_POINT('',(80.,72.,17.2));
#36670=CARTESIAN_POINT('',(80.5,72.5,17.2));
#36671=CARTESIAN_POINT('',(80.,72.,17.2));
#36672=CARTESIAN_POINT('',(80.5,72.5,9.75));
#36673=CARTESIAN_POINT('',(80.,72.,9.75));
#36674=CARTESIAN_POINT('Origin',(79.2,72.25,17.2));
#36675=CARTESIAN_POINT('Origin',(79.2,72.,17.2));
#36676=CARTESIAN_POINT('',(79.2,72.5,18.5));
#36677=CARTESIAN_POINT('',(79.2,72.,18.));
#36678=CARTESIAN_POINT('Origin',(79.2,72.5,17.2));
#36679=CARTESIAN_POINT('Origin',(70.5,72.25,18.25));
#36680=CARTESIAN_POINT('',(42.8,72.5,18.5));
#36681=CARTESIAN_POINT('',(42.8,72.,18.));
#36682=CARTESIAN_POINT('',(70.5,72.5,18.5));
#36683=CARTESIAN_POINT('Origin',(42.8,72.25,17.2));
#36684=CARTESIAN_POINT('',(41.5,72.5,17.2));
#36685=CARTESIAN_POINT('',(42.,72.,17.2));
#36686=CARTESIAN_POINT('Origin',(42.8,72.5,17.2));
#36687=CARTESIAN_POINT('Origin',(41.75,72.25,15.75));
#36688=CARTESIAN_POINT('',(41.5,72.5,6.8));
#36689=CARTESIAN_POINT('',(42.,72.,6.8));
#36690=CARTESIAN_POINT('',(41.5,72.5,15.75));
#36691=CARTESIAN_POINT('Origin',(41.2,72.25,6.8));
#36692=CARTESIAN_POINT('',(41.2,72.5,6.5));
#36693=CARTESIAN_POINT('',(41.2,72.,6.));
#36694=CARTESIAN_POINT('Origin',(41.2,72.5,6.8));
#36695=CARTESIAN_POINT('Origin',(51.5,72.25,6.25));
#36696=CARTESIAN_POINT('',(39.8,72.5,6.5));
#36697=CARTESIAN_POINT('',(39.8,72.,6.));
#36698=CARTESIAN_POINT('',(51.5,72.5,6.5));
#36699=CARTESIAN_POINT('Origin',(39.8,72.25,6.8));
#36700=CARTESIAN_POINT('',(39.5,72.5,6.8));
#36701=CARTESIAN_POINT('',(39.,72.,6.8));
#36702=CARTESIAN_POINT('Origin',(39.8,72.5,6.8));
#36703=CARTESIAN_POINT('Origin',(39.25,72.25,9.75));
#36704=CARTESIAN_POINT('',(39.5,72.5,20.2));
#36705=CARTESIAN_POINT('',(39.,72.,20.2));
#36706=CARTESIAN_POINT('',(39.5,72.5,9.75));
#36707=CARTESIAN_POINT('Origin',(39.8,72.25,20.2));
#36708=CARTESIAN_POINT('Origin',(39.8,72.5,20.2));
#36709=CARTESIAN_POINT('Origin',(79.2,-72.5,17.2));
#36710=CARTESIAN_POINT('',(80.,-72.5,17.2));
#36711=CARTESIAN_POINT('Origin',(80.,-72.5,6.));
#36712=CARTESIAN_POINT('',(80.,-72.5,6.8));
#36713=CARTESIAN_POINT('Origin',(80.8,-72.5,6.8));
#36714=CARTESIAN_POINT('',(80.8,-72.5,6.));
#36715=CARTESIAN_POINT('Origin',(83.,-72.5,6.));
#36716=CARTESIAN_POINT('',(82.2,-72.5,6.));
#36717=CARTESIAN_POINT('Origin',(82.2,-72.5,6.8));
#36718=CARTESIAN_POINT('',(83.,-72.5,6.8));
#36719=CARTESIAN_POINT('Origin',(83.,-72.5,21.));
#36720=CARTESIAN_POINT('',(83.,-72.5,20.2));
#36721=CARTESIAN_POINT('Origin',(82.2,-72.5,20.2));
#36722=CARTESIAN_POINT('Origin',(61.,72.5,13.5));
#36723=CARTESIAN_POINT('Origin',(61.,66.,20.75));
#36724=CARTESIAN_POINT('',(57.25,66.,20.75));
#36725=CARTESIAN_POINT('Origin',(61.,-66.,20.75));
#36726=CARTESIAN_POINT('',(57.25,-66.,20.75));
#36727=CARTESIAN_POINT('Origin',(61.,-52.5,21.));
#36728=CARTESIAN_POINT('',(56.5,-52.5,21.));
#36729=CARTESIAN_POINT('Origin',(61.,25.,21.));
#36730=CARTESIAN_POINT('',(56.5,25.,21.));
#36731=CARTESIAN_POINT('Origin',(61.,-25.,21.));
#36732=CARTESIAN_POINT('',(56.5,-25.,21.));
#36733=CARTESIAN_POINT('Origin',(61.,52.5,21.));
#36734=CARTESIAN_POINT('',(56.5,52.5,21.));
#56612=UNCERTAINTY_MEASURE_WITH_UNIT(LENGTH_MEASURE(0.01),#56640,
'DISTANCE_ACCURACY_VALUE',
'Maximum model space distance between geometric entities at asserted c
onnectivities');
#56617=UNCERTAINTY_MEASURE_WITH_UNIT(LENGTH_MEASURE(0.01),#56640,
'DISTANCE_ACCURACY_VALUE',
'Maximum model space distance between geometric entities at asserted c
onnectivities');
#56634=(
GEOMETRIC_REPRESENTATION_CONTEXT(3)
GLOBAL_UNCERTAINTY_ASSIGNED_CONTEXT((#56612))
GLOBAL_UNIT_ASSIGNED_CONTEXT((#56640,#56642,#56643))
REPRESENTATION_CONTEXT('','3D')
);
#56639=(
GEOMETRIC_REPRESENTATION_CONTEXT(3)
GLOBAL_UNCERTAINTY_ASSIGNED_CONTEXT((#56617))
GLOBAL_UNIT_ASSIGNED_CONTEXT((#56640,#56642,#56643))
REPRESENTATION_CONTEXT('','3D')
);
#56640=(
LENGTH_UNIT()
NAMED_UNIT(*)
SI_UNIT(.MILLI.,.METRE.)
);
#56642=(
NAMED_UNIT(*)
PLANE_ANGLE_UNIT()
SI_UNIT($,.RADIAN.)
);
#56643=(
NAMED_UNIT(*)
SI_UNIT($,.STERADIAN.)
SOLID_ANGLE_UNIT()
);
#56660=SHAPE_DEFINITION_REPRESENTATION(#56681,#56760);
#56681=PRODUCT_DEFINITION_SHAPE('',$,#56782);
#56760=SHAPE_REPRESENTATION('',(#18218),#56634);
#56765=PRODUCT_DEFINITION_CONTEXT('part definition',#56830,'design');
#56782=PRODUCT_DEFINITION('2026-10-26-00-02-50-838','14_Base_Channel',#56803,
#56765);
#56803=PRODUCT_DEFINITION_FORMATION('',$,#56848);
#56830=APPLICATION_CONTEXT(
'Core Data for Automotive Mechanical Design Process');
#56831=PRODUCT_CONTEXT('part definition',#56830,'mechanical');
#56848=PRODUCT('2026-10-26-00-02-50-838','14_Base_Channel',$,(#56831));
#56888=COLOUR_RGB('Dark Blue',0.08,0.2,0.34);
#56889=FILL_AREA_STYLE_COLOUR('',#56888);
#56890=FILL_AREA_STYLE('',(#56889));
#56891=SURFACE_STYLE_FILL_AREA(#56890);
#56892=SURFACE_SIDE_STYLE('',(#56891));
#56893=SURFACE_STYLE_USAGE(.BOTH.,#56892);
#56894=PRESENTATION_STYLE_ASSIGNMENT((#56893));
ENDSEC;
END-ISO-10303-21;
